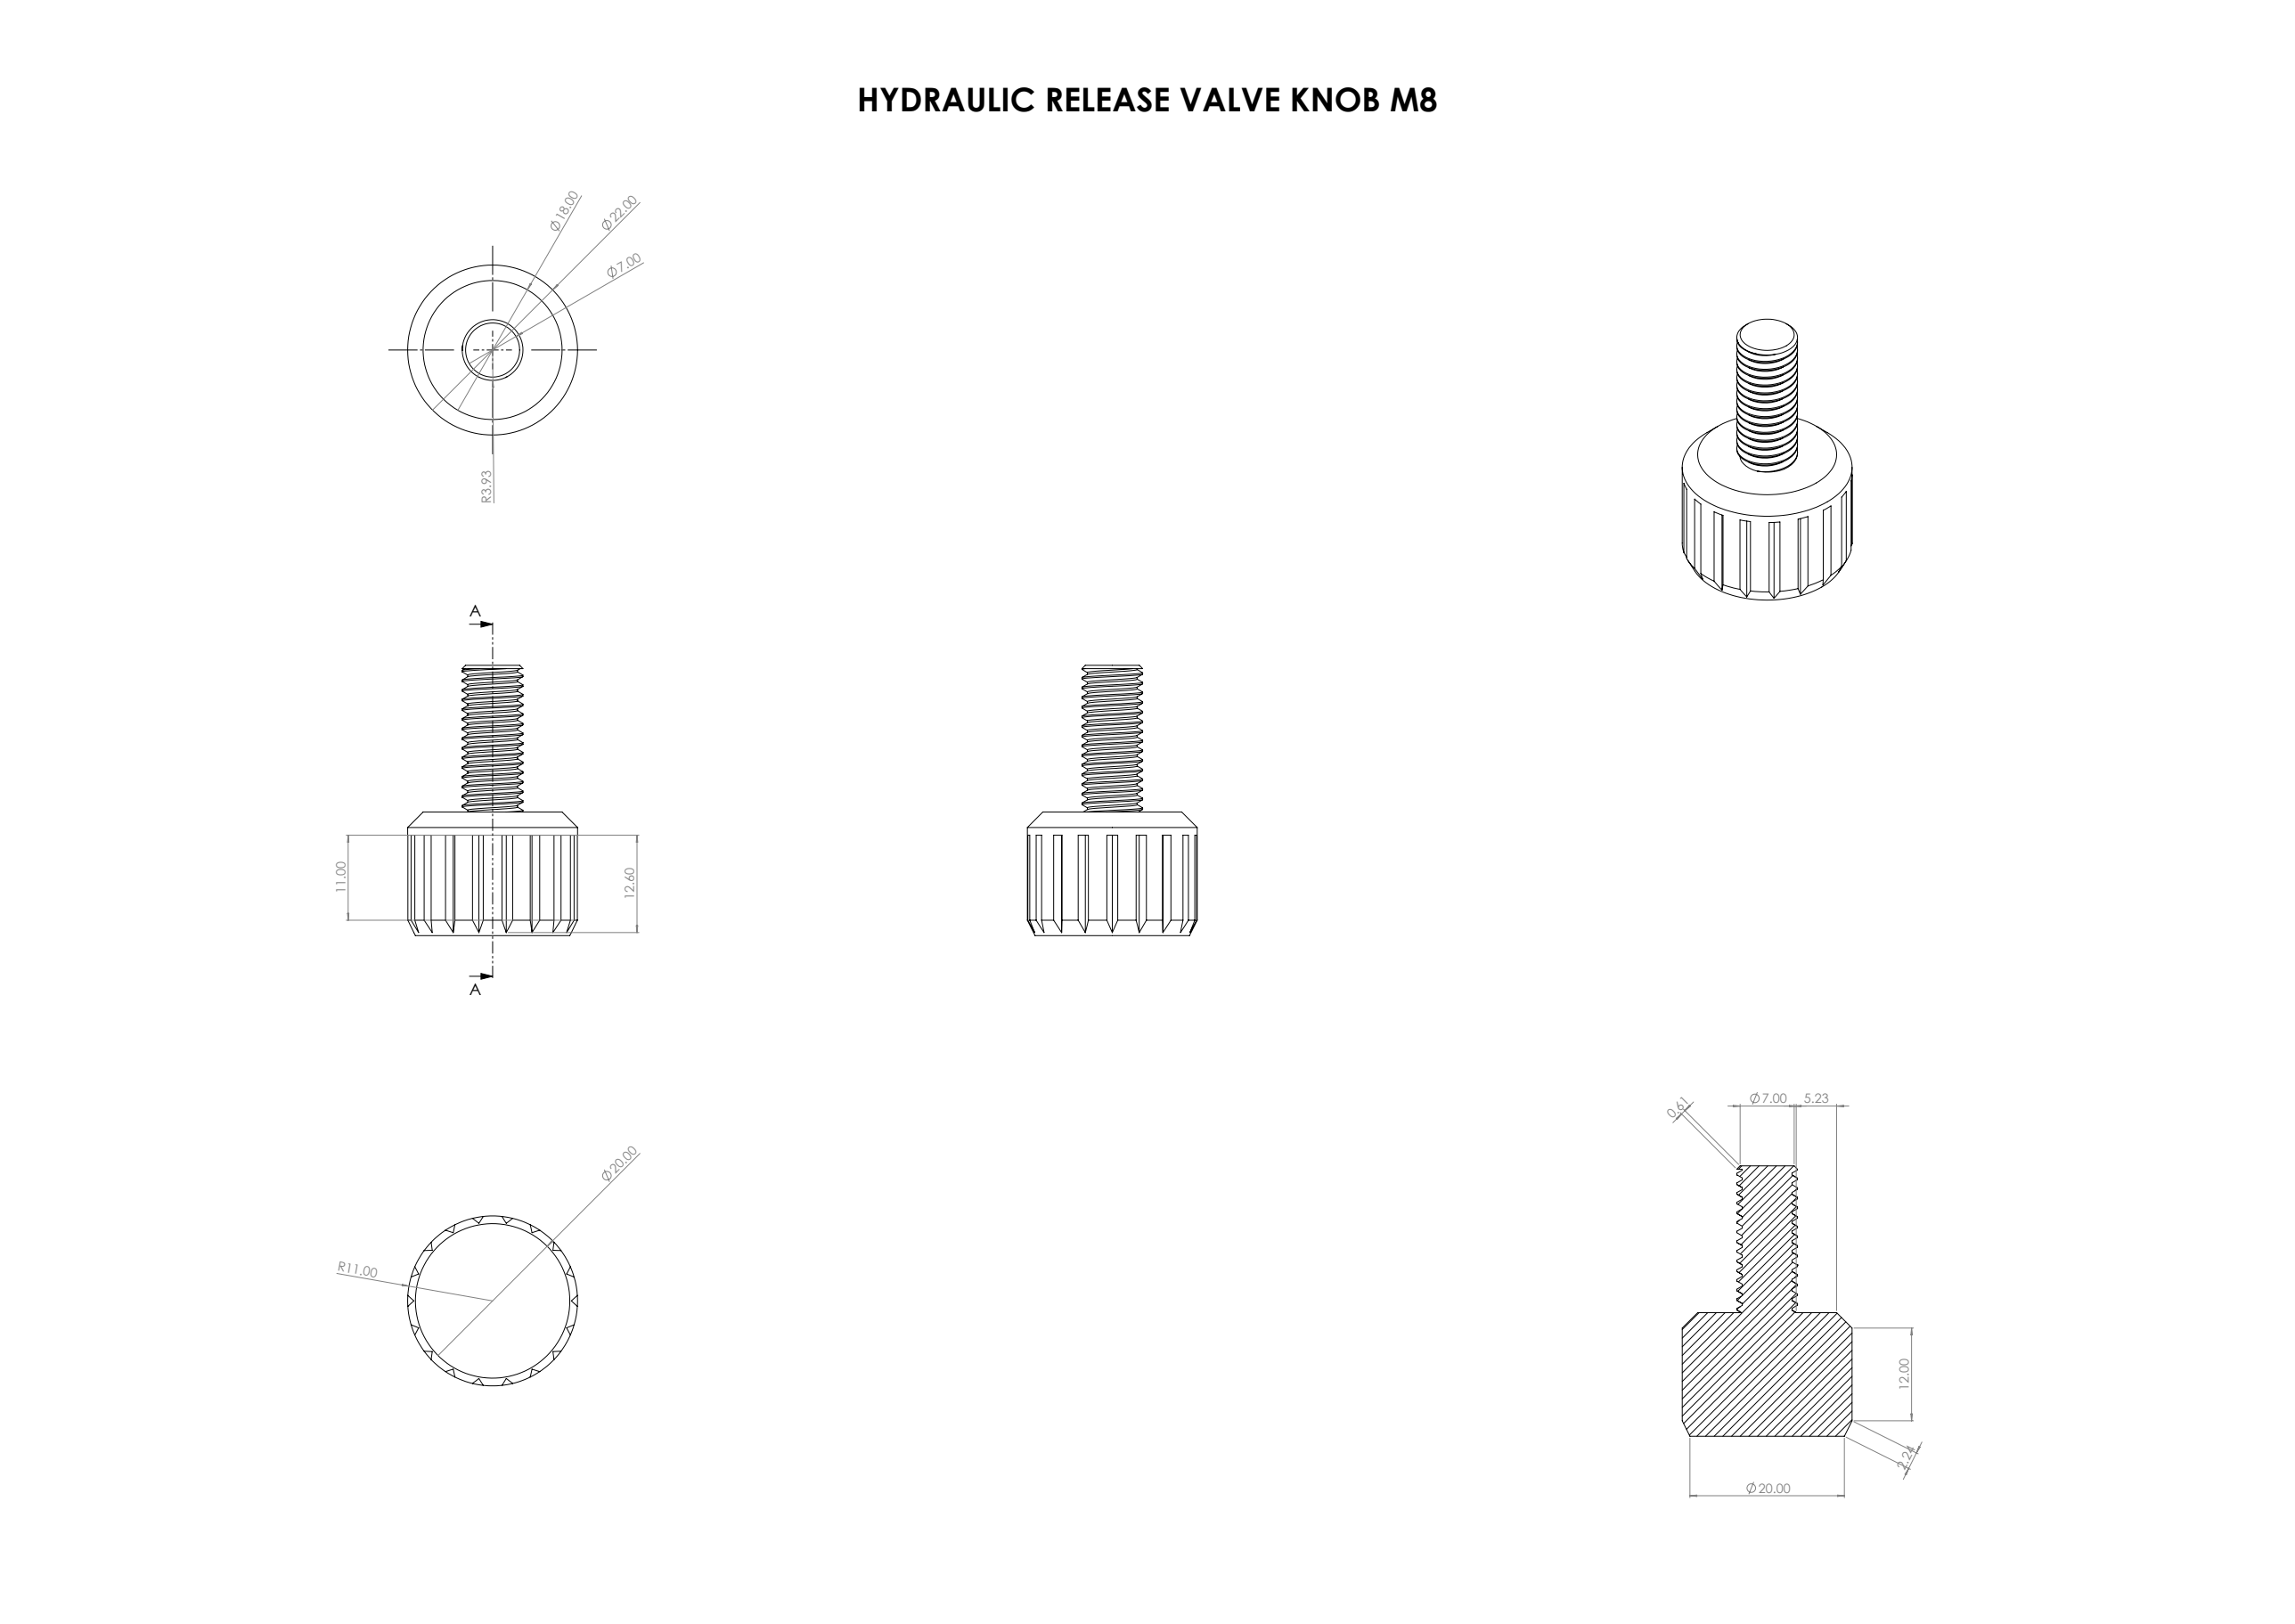
ISO-10303-21;
HEADER;
/* Generated by software containing ST-Developer
 * from STEP Tools, Inc. (www.steptools.com) 
 */

FILE_DESCRIPTION(
/* description */ (''),
/* implementation_level */ '2;1');

FILE_NAME(
/* name */ '12_Hydraulic_Release_Valve_Knob_M8.step',
/* time_stamp */ '2026-10-20T10:03:03-07:00',
/* author */ (''),
/* organization */ (''),
/* preprocessor_version */ 'ST-DEVELOPER v20.2',
/* originating_system */ 'Autodesk Translation Framework v15.15.0.0',
/* authorisation */ '');

FILE_SCHEMA (('AUTOMOTIVE_DESIGN { 1 0 10303 214 3 1 1 }'));
ENDSEC;

DATA;
#10=MECHANICAL_DESIGN_GEOMETRIC_PRESENTATION_REPRESENTATION('',(#530),#71492);
#319=(
BOUNDED_CURVE()
B_SPLINE_CURVE(2,(#47148,#47149,#47150),.UNSPECIFIED.,.F.,.F.)
B_SPLINE_CURVE_WITH_KNOTS((3,3),(0.0512618960218088,0.239747982802954),
 .UNSPECIFIED.)
CURVE()
GEOMETRIC_REPRESENTATION_ITEM()
RATIONAL_B_SPLINE_CURVE((1.0006680999084,1.00156232618943,1.))
REPRESENTATION_ITEM('')
);
#320=(
BOUNDED_CURVE()
B_SPLINE_CURVE(2,(#47162,#47163,#47164),.UNSPECIFIED.,.F.,.F.)
B_SPLINE_CURVE_WITH_KNOTS((3,3),(0.,0.18848608678106),.UNSPECIFIED.)
CURVE()
GEOMETRIC_REPRESENTATION_ITEM()
RATIONAL_B_SPLINE_CURVE((1.,1.0015623261938,1.00066809991027))
REPRESENTATION_ITEM('')
);
#321=(
BOUNDED_CURVE()
B_SPLINE_CURVE(2,(#47169,#47170,#47171),.UNSPECIFIED.,.F.,.F.)
B_SPLINE_CURVE_WITH_KNOTS((3,3),(0.0512618960217405,0.239747982802953),
 .UNSPECIFIED.)
CURVE()
GEOMETRIC_REPRESENTATION_ITEM()
RATIONAL_B_SPLINE_CURVE((1.00066809990968,1.00156232619242,1.))
REPRESENTATION_ITEM('')
);
#322=(
BOUNDED_CURVE()
B_SPLINE_CURVE(2,(#47183,#47184,#47185),.UNSPECIFIED.,.F.,.F.)
B_SPLINE_CURVE_WITH_KNOTS((3,3),(0.,0.188486086781626),.UNSPECIFIED.)
CURVE()
GEOMETRIC_REPRESENTATION_ITEM()
RATIONAL_B_SPLINE_CURVE((1.,1.00156232620375,1.00066809991451))
REPRESENTATION_ITEM('')
);
#323=(
BOUNDED_CURVE()
B_SPLINE_CURVE(2,(#47190,#47191,#47192),.UNSPECIFIED.,.F.,.F.)
B_SPLINE_CURVE_WITH_KNOTS((3,3),(0.051261896021783,0.239747982802949),
 .UNSPECIFIED.)
CURVE()
GEOMETRIC_REPRESENTATION_ITEM()
RATIONAL_B_SPLINE_CURVE((1.0006680999091,1.00156232619108,1.))
REPRESENTATION_ITEM('')
);
#324=(
BOUNDED_CURVE()
B_SPLINE_CURVE(2,(#47204,#47205,#47206),.UNSPECIFIED.,.F.,.F.)
B_SPLINE_CURVE_WITH_KNOTS((3,3),(0.,0.188486086780641),.UNSPECIFIED.)
CURVE()
GEOMETRIC_REPRESENTATION_ITEM()
RATIONAL_B_SPLINE_CURVE((1.,1.00156232617076,1.00066809990042))
REPRESENTATION_ITEM('')
);
#325=(
BOUNDED_CURVE()
B_SPLINE_CURVE(2,(#47211,#47212,#47213),.UNSPECIFIED.,.F.,.F.)
B_SPLINE_CURVE_WITH_KNOTS((3,3),(0.0512618960212928,0.239747982802966),
 .UNSPECIFIED.)
CURVE()
GEOMETRIC_REPRESENTATION_ITEM()
RATIONAL_B_SPLINE_CURVE((1.00066809991313,1.0015623262005,1.))
REPRESENTATION_ITEM('')
);
#326=(
BOUNDED_CURVE()
B_SPLINE_CURVE(2,(#47225,#47226,#47227),.UNSPECIFIED.,.F.,.F.)
B_SPLINE_CURVE_WITH_KNOTS((3,3),(0.,0.18848608678103),.UNSPECIFIED.)
CURVE()
GEOMETRIC_REPRESENTATION_ITEM()
RATIONAL_B_SPLINE_CURVE((1.,1.00156232618489,1.00066809990646))
REPRESENTATION_ITEM('')
);
#327=(
BOUNDED_CURVE()
B_SPLINE_CURVE(2,(#47232,#47233,#47234),.UNSPECIFIED.,.F.,.F.)
B_SPLINE_CURVE_WITH_KNOTS((3,3),(0.0512618960214512,0.239747982802948),
 .UNSPECIFIED.)
CURVE()
GEOMETRIC_REPRESENTATION_ITEM()
RATIONAL_B_SPLINE_CURVE((1.00066809991422,1.00156232620306,1.))
REPRESENTATION_ITEM('')
);
#328=(
BOUNDED_CURVE()
B_SPLINE_CURVE(2,(#47246,#47247,#47248),.UNSPECIFIED.,.F.,.F.)
B_SPLINE_CURVE_WITH_KNOTS((3,3),(0.,0.188486086781497),.UNSPECIFIED.)
CURVE()
GEOMETRIC_REPRESENTATION_ITEM()
RATIONAL_B_SPLINE_CURVE((1.,1.00156232620306,1.00066809991422))
REPRESENTATION_ITEM('')
);
#329=(
BOUNDED_CURVE()
B_SPLINE_CURVE(2,(#47253,#47254,#47255),.UNSPECIFIED.,.F.,.F.)
B_SPLINE_CURVE_WITH_KNOTS((3,3),(0.0512618960218087,0.239747982802954),
 .UNSPECIFIED.)
CURVE()
GEOMETRIC_REPRESENTATION_ITEM()
RATIONAL_B_SPLINE_CURVE((1.0006680999084,1.00156232618943,1.))
REPRESENTATION_ITEM('')
);
#330=(
BOUNDED_CURVE()
B_SPLINE_CURVE(2,(#47267,#47268,#47269),.UNSPECIFIED.,.F.,.F.)
B_SPLINE_CURVE_WITH_KNOTS((3,3),(0.,0.188486086780909),.UNSPECIFIED.)
CURVE()
GEOMETRIC_REPRESENTATION_ITEM()
RATIONAL_B_SPLINE_CURVE((1.,1.00156232618876,1.00066809990812))
REPRESENTATION_ITEM('')
);
#331=(
BOUNDED_CURVE()
B_SPLINE_CURVE(2,(#47274,#47275,#47276),.UNSPECIFIED.,.F.,.F.)
B_SPLINE_CURVE_WITH_KNOTS((3,3),(0.0512618960214397,0.239747982802953),
 .UNSPECIFIED.)
CURVE()
GEOMETRIC_REPRESENTATION_ITEM()
RATIONAL_B_SPLINE_CURVE((1.00066809991433,1.00156232620331,1.))
REPRESENTATION_ITEM('')
);
#332=(
BOUNDED_CURVE()
B_SPLINE_CURVE(2,(#47288,#47289,#47290),.UNSPECIFIED.,.F.,.F.)
B_SPLINE_CURVE_WITH_KNOTS((3,3),(0.,0.188486086781649),.UNSPECIFIED.)
CURVE()
GEOMETRIC_REPRESENTATION_ITEM()
RATIONAL_B_SPLINE_CURVE((1.,1.00156232620001,1.00066809991291))
REPRESENTATION_ITEM('')
);
#333=(
BOUNDED_CURVE()
B_SPLINE_CURVE(2,(#47295,#47296,#47297),.UNSPECIFIED.,.F.,.F.)
B_SPLINE_CURVE_WITH_KNOTS((3,3),(0.0512618960219227,0.239747982802949),
 .UNSPECIFIED.)
CURVE()
GEOMETRIC_REPRESENTATION_ITEM()
RATIONAL_B_SPLINE_CURVE((1.00066809990695,1.00156232618604,1.))
REPRESENTATION_ITEM('')
);
#334=(
BOUNDED_CURVE()
B_SPLINE_CURVE(2,(#47309,#47310,#47311),.UNSPECIFIED.,.F.,.F.)
B_SPLINE_CURVE_WITH_KNOTS((3,3),(0.,0.188486086780641),.UNSPECIFIED.)
CURVE()
GEOMETRIC_REPRESENTATION_ITEM()
RATIONAL_B_SPLINE_CURVE((1.,1.00156232617076,1.00066809990042))
REPRESENTATION_ITEM('')
);
#335=(
BOUNDED_CURVE()
B_SPLINE_CURVE(2,(#47316,#47317,#47318),.UNSPECIFIED.,.F.,.F.)
B_SPLINE_CURVE_WITH_KNOTS((3,3),(0.0512618960215005,0.239747982802966),
 .UNSPECIFIED.)
CURVE()
GEOMETRIC_REPRESENTATION_ITEM()
RATIONAL_B_SPLINE_CURVE((1.00066809990987,1.00156232619288,1.))
REPRESENTATION_ITEM('')
);
#336=(
BOUNDED_CURVE()
B_SPLINE_CURVE(2,(#47330,#47331,#47332),.UNSPECIFIED.,.F.,.F.)
B_SPLINE_CURVE_WITH_KNOTS((3,3),(0.,0.188486086781019),.UNSPECIFIED.)
CURVE()
GEOMETRIC_REPRESENTATION_ITEM()
RATIONAL_B_SPLINE_CURVE((1.,1.00156232618454,1.00066809990631))
REPRESENTATION_ITEM('')
);
#337=(
BOUNDED_CURVE()
B_SPLINE_CURVE(2,(#47337,#47338,#47339),.UNSPECIFIED.,.F.,.F.)
B_SPLINE_CURVE_WITH_KNOTS((3,3),(0.0512618960218745,0.239747982802939),
 .UNSPECIFIED.)
CURVE()
GEOMETRIC_REPRESENTATION_ITEM()
RATIONAL_B_SPLINE_CURVE((1.00066809991027,1.0015623261938,1.))
REPRESENTATION_ITEM('')
);
#338=(
BOUNDED_CURVE()
B_SPLINE_CURVE(2,(#47351,#47352,#47353),.UNSPECIFIED.,.F.,.F.)
B_SPLINE_CURVE_WITH_KNOTS((3,3),(0.,0.188486086781156),.UNSPECIFIED.)
CURVE()
GEOMETRIC_REPRESENTATION_ITEM()
RATIONAL_B_SPLINE_CURVE((1.,1.00156232618832,1.00066809990792))
REPRESENTATION_ITEM('')
);
#339=(
BOUNDED_CURVE()
B_SPLINE_CURVE(2,(#47358,#47359,#47360),.UNSPECIFIED.,.F.,.F.)
B_SPLINE_CURVE_WITH_KNOTS((3,3),(0.0512618960213807,0.239747982802952),
 .UNSPECIFIED.)
CURVE()
GEOMETRIC_REPRESENTATION_ITEM()
RATIONAL_B_SPLINE_CURVE((1.00066809991545,1.00156232620592,1.))
REPRESENTATION_ITEM('')
);
#340=(
BOUNDED_CURVE()
B_SPLINE_CURVE(2,(#47372,#47373,#47374),.UNSPECIFIED.,.F.,.F.)
B_SPLINE_CURVE_WITH_KNOTS((3,3),(0.,0.188486086781477),.UNSPECIFIED.)
CURVE()
GEOMETRIC_REPRESENTATION_ITEM()
RATIONAL_B_SPLINE_CURVE((1.,1.0015623262088,1.00066809991668))
REPRESENTATION_ITEM('')
);
#341=(
BOUNDED_CURVE()
B_SPLINE_CURVE(2,(#47379,#47380,#47381),.UNSPECIFIED.,.F.,.F.)
B_SPLINE_CURVE_WITH_KNOTS((3,3),(0.0512618960223282,0.239747982802951),
 .UNSPECIFIED.)
CURVE()
GEOMETRIC_REPRESENTATION_ITEM()
RATIONAL_B_SPLINE_CURVE((1.00066809990016,1.00156232617014,1.))
REPRESENTATION_ITEM('')
);
#342=(
BOUNDED_CURVE()
B_SPLINE_CURVE(2,(#47393,#47394,#47395),.UNSPECIFIED.,.F.,.F.)
B_SPLINE_CURVE_WITH_KNOTS((3,3),(0.,0.188486086781308),.UNSPECIFIED.)
CURVE()
GEOMETRIC_REPRESENTATION_ITEM()
RATIONAL_B_SPLINE_CURVE((1.,1.00156232619586,1.00066809991115))
REPRESENTATION_ITEM('')
);
#343=(
BOUNDED_CURVE()
B_SPLINE_CURVE(2,(#47400,#47401,#47402),.UNSPECIFIED.,.F.,.F.)
B_SPLINE_CURVE_WITH_KNOTS((3,3),(0.051261896021939,0.239747982802949),
 .UNSPECIFIED.)
CURVE()
GEOMETRIC_REPRESENTATION_ITEM()
RATIONAL_B_SPLINE_CURVE((1.00066809990618,1.00156232618425,1.))
REPRESENTATION_ITEM('')
);
#344=(
BOUNDED_CURVE()
B_SPLINE_CURVE(2,(#47414,#47415,#47416),.UNSPECIFIED.,.F.,.F.)
B_SPLINE_CURVE_WITH_KNOTS((3,3),(0.,0.188486086781416),.UNSPECIFIED.)
CURVE()
GEOMETRIC_REPRESENTATION_ITEM()
RATIONAL_B_SPLINE_CURVE((1.,1.0015623261913,1.0006680999092))
REPRESENTATION_ITEM('')
);
#345=(
BOUNDED_CURVE()
B_SPLINE_CURVE(2,(#47421,#47422,#47423),.UNSPECIFIED.,.F.,.F.)
B_SPLINE_CURVE_WITH_KNOTS((3,3),(0.0512618960214561,0.239747982802948),
 .UNSPECIFIED.)
CURVE()
GEOMETRIC_REPRESENTATION_ITEM()
RATIONAL_B_SPLINE_CURVE((1.00066809991424,1.00156232620311,1.))
REPRESENTATION_ITEM('')
);
#346=(
BOUNDED_CURVE()
B_SPLINE_CURVE(2,(#47437,#47438,#47439),.UNSPECIFIED.,.F.,.F.)
B_SPLINE_CURVE_WITH_KNOTS((3,3),(0.,0.188486086781106),.UNSPECIFIED.)
CURVE()
GEOMETRIC_REPRESENTATION_ITEM()
RATIONAL_B_SPLINE_CURVE((1.,1.00156232618923,1.00066809990831))
REPRESENTATION_ITEM('')
);
#347=(
BOUNDED_CURVE()
B_SPLINE_CURVE(2,(#47444,#47445,#47446),.UNSPECIFIED.,.F.,.F.)
B_SPLINE_CURVE_WITH_KNOTS((3,3),(0.0512618960218789,0.239747982802938),
 .UNSPECIFIED.)
CURVE()
GEOMETRIC_REPRESENTATION_ITEM()
RATIONAL_B_SPLINE_CURVE((1.00066809991027,1.0015623261938,1.))
REPRESENTATION_ITEM('')
);
#348=(
BOUNDED_CURVE()
B_SPLINE_CURVE(2,(#47458,#47459,#47460),.UNSPECIFIED.,.F.,.F.)
B_SPLINE_CURVE_WITH_KNOTS((3,3),(0.,0.188486086781156),.UNSPECIFIED.)
CURVE()
GEOMETRIC_REPRESENTATION_ITEM()
RATIONAL_B_SPLINE_CURVE((1.,1.00156232618832,1.00066809990792))
REPRESENTATION_ITEM('')
);
#349=(
BOUNDED_CURVE()
B_SPLINE_CURVE(2,(#47465,#47466,#47467),.UNSPECIFIED.,.F.,.F.)
B_SPLINE_CURVE_WITH_KNOTS((3,3),(0.0512618960211266,0.239747982802957),
 .UNSPECIFIED.)
CURVE()
GEOMETRIC_REPRESENTATION_ITEM()
RATIONAL_B_SPLINE_CURVE((1.00066809991756,1.00156232621087,1.))
REPRESENTATION_ITEM('')
);
#350=(
BOUNDED_CURVE()
B_SPLINE_CURVE(2,(#47479,#47480,#47481),.UNSPECIFIED.,.F.,.F.)
B_SPLINE_CURVE_WITH_KNOTS((3,3),(0.,0.188486086781475),.UNSPECIFIED.)
CURVE()
GEOMETRIC_REPRESENTATION_ITEM()
RATIONAL_B_SPLINE_CURVE((1.,1.0015623262088,1.00066809991668))
REPRESENTATION_ITEM('')
);
#351=(
BOUNDED_CURVE()
B_SPLINE_CURVE(2,(#47486,#47487,#47488),.UNSPECIFIED.,.F.,.F.)
B_SPLINE_CURVE_WITH_KNOTS((3,3),(0.0512618960222505,0.239747982802951),
 .UNSPECIFIED.)
CURVE()
GEOMETRIC_REPRESENTATION_ITEM()
RATIONAL_B_SPLINE_CURVE((1.00066809990131,1.00156232617284,1.))
REPRESENTATION_ITEM('')
);
#352=(
BOUNDED_CURVE()
B_SPLINE_CURVE(2,(#47500,#47501,#47502),.UNSPECIFIED.,.F.,.F.)
B_SPLINE_CURVE_WITH_KNOTS((3,3),(0.,0.188486086781171),.UNSPECIFIED.)
CURVE()
GEOMETRIC_REPRESENTATION_ITEM()
RATIONAL_B_SPLINE_CURVE((1.,1.00156232619143,1.00066809990925))
REPRESENTATION_ITEM('')
);
#353=(
BOUNDED_CURVE()
B_SPLINE_CURVE(2,(#47507,#47508,#47509),.UNSPECIFIED.,.F.,.F.)
B_SPLINE_CURVE_WITH_KNOTS((3,3),(0.0512618960219306,0.239747982802949),
 .UNSPECIFIED.)
CURVE()
GEOMETRIC_REPRESENTATION_ITEM()
RATIONAL_B_SPLINE_CURVE((1.00066809990631,1.00156232618454,1.))
REPRESENTATION_ITEM('')
);
#354=(
BOUNDED_CURVE()
B_SPLINE_CURVE(2,(#47521,#47522,#47523),.UNSPECIFIED.,.F.,.F.)
B_SPLINE_CURVE_WITH_KNOTS((3,3),(0.,0.188486086781674),.UNSPECIFIED.)
CURVE()
GEOMETRIC_REPRESENTATION_ITEM()
RATIONAL_B_SPLINE_CURVE((1.,1.0015623262005,1.00066809991312))
REPRESENTATION_ITEM('')
);
#388=SHAPE_REPRESENTATION_RELATIONSHIP('SRR','None',#71609,#407);
#407=ADVANCED_BREP_SHAPE_REPRESENTATION('',(#426),#71479);
#426=MANIFOLD_SOLID_BREP('Release knob',#28465);
#530=STYLED_ITEM('',(#71873),#426);
#810=B_SPLINE_CURVE_WITH_KNOTS('',3,(#46072,#46073,#46074,#46075,#46076,
#46077,#46078,#46079,#46080,#46081),.UNSPECIFIED.,.F.,.F.,(4,3,3,4),(-4.09274904019441,
-3.97454678650995,-2.98091008988247,-2.06120159751572),.UNSPECIFIED.);
#811=B_SPLINE_CURVE_WITH_KNOTS('',3,(#46084,#46085,#46086,#46087,#46088,
#46089,#46090,#46091,#46092,#46093),.UNSPECIFIED.,.F.,.F.,(4,3,3,4),(0.,
0.496818348313743,0.993636696627499,1.11004521091142),.UNSPECIFIED.);
#812=B_SPLINE_CURVE_WITH_KNOTS('',3,(#46098,#46099,#46100,#46101,#46102,
#46103,#46104,#46105,#46106,#46107,#46108,#46109,#46110,#46111,#46112,#46113,
#46114,#46115,#46116,#46117,#46118,#46119),.UNSPECIFIED.,.F.,.F.,(4,3,3,
3,3,3,3,4),(-10.375934347374,-9.93636696627486,-8.94273026964737,-7.94909357301989,
-6.9554568763924,-5.96182017976492,-4.96818348313743,-4.09274904019441),
 .UNSPECIFIED.);
#813=B_SPLINE_CURVE_WITH_KNOTS('',3,(#46120,#46121,#46122,#46123,#46124,
#46125,#46126,#46127,#46128,#46129,#46130,#46131,#46132,#46133,#46134,#46135,
#46136,#46137,#46138,#46139,#46140,#46141),.UNSPECIFIED.,.F.,.F.,(4,3,3,
3,3,3,3,4),(1.11004521091142,1.98727339325499,2.98091008988248,3.97454678650997,
4.96818348313745,5.96182017976494,6.95545687639243,7.393230518091),
 .UNSPECIFIED.);
#814=B_SPLINE_CURVE_WITH_KNOTS('',3,(#46146,#46147,#46148,#46149,#46150,
#46151,#46152,#46153,#46154,#46155,#46156,#46157,#46158,#46159,#46160,#46161,
#46162,#46163,#46164,#46165,#46166,#46167),.UNSPECIFIED.,.F.,.F.,(4,3,3,
3,3,3,3,4),(-16.6591196545536,-15.8981871460398,-14.9045504494123,-13.9109137527848,
-12.9172770561573,-11.9236403595298,-10.9300036629023,-10.375934347374),
 .UNSPECIFIED.);
#815=B_SPLINE_CURVE_WITH_KNOTS('',3,(#46168,#46169,#46170,#46171,#46172,
#46173,#46174,#46175,#46176,#46177,#46178,#46179,#46180,#46181,#46182,#46183,
#46184,#46185,#46186,#46187,#46188,#46189),.UNSPECIFIED.,.F.,.F.,(4,3,3,
3,3,3,3,4),(7.393230518091,7.94909357301991,8.94273026964739,9.93636696627487,
10.9300036629024,11.9236403595298,12.9172770561573,13.6764158252706),
 .UNSPECIFIED.);
#816=B_SPLINE_CURVE_WITH_KNOTS('',3,(#46194,#46195,#46196,#46197,#46198,
#46199,#46200,#46201,#46202,#46203,#46204,#46205,#46206,#46207,#46208,#46209,
#46210,#46211,#46212,#46213,#46214,#46215,#46216,#46217,#46218),
 .UNSPECIFIED.,.F.,.F.,(4,3,3,3,3,3,3,3,4),(-22.9423049617332,-22.8536440224322,
-21.8600073258047,-20.8663706291772,-19.8727339325497,-18.8790972359222,
-17.8854605392947,-16.8918238426673,-16.6591196545536),.UNSPECIFIED.);
#817=B_SPLINE_CURVE_WITH_KNOTS('',3,(#46219,#46220,#46221,#46222,#46223,
#46224,#46225,#46226,#46227,#46228,#46229,#46230,#46231,#46232,#46233,#46234,
#46235,#46236,#46237,#46238,#46239,#46240,#46241,#46242,#46243),
 .UNSPECIFIED.,.F.,.F.,(4,3,3,3,3,3,3,3,4),(13.6764158252706,13.9109137527848,
14.9045504494123,15.8981871460398,16.8918238426673,17.8854605392947,18.8790972359222,
19.8727339325497,19.9596011324502),.UNSPECIFIED.);
#818=B_SPLINE_CURVE_WITH_KNOTS('',3,(#46248,#46249,#46250,#46251,#46252,
#46253,#46254,#46255,#46256,#46257,#46258,#46259,#46260,#46261,#46262,#46263,
#46264,#46265,#46266,#46267,#46268,#46269),.UNSPECIFIED.,.F.,.F.,(4,3,3,
3,3,3,3,4),(-29.2254902689127,-28.8154642021971,-27.8218275055696,-26.8281908089421,
-25.8345541123146,-24.8409174156871,-23.8472807190597,-22.9423049617332),
 .UNSPECIFIED.);
#819=B_SPLINE_CURVE_WITH_KNOTS('',3,(#46270,#46271,#46272,#46273,#46274,
#46275,#46276,#46277,#46278,#46279,#46280,#46281,#46282,#46283,#46284,#46285,
#46286,#46287,#46288,#46289,#46290,#46291),.UNSPECIFIED.,.F.,.F.,(4,3,3,
3,3,3,3,4),(19.9596011324502,20.8663706291772,21.8600073258047,22.8536440224322,
23.8472807190597,24.8409174156871,25.8345541123146,26.2427864396298),
 .UNSPECIFIED.);
#820=B_SPLINE_CURVE_WITH_KNOTS('',3,(#46296,#46297,#46298,#46299,#46300,
#46301,#46302,#46303,#46304,#46305,#46306,#46307,#46308,#46309,#46310,#46311,
#46312,#46313,#46314,#46315,#46316,#46317),.UNSPECIFIED.,.F.,.F.,(4,3,3,
3,3,3,3,4),(-35.5086755760923,-34.777284381962,-33.7836476853345,-32.790010988707,
-31.7963742920795,-30.802737595452,-29.8091008988246,-29.2254902689127),
 .UNSPECIFIED.);
#821=B_SPLINE_CURVE_WITH_KNOTS('',3,(#46318,#46319,#46320,#46321,#46322,
#46323,#46324,#46325,#46326,#46327,#46328,#46329,#46330,#46331,#46332,#46333,
#46334,#46335,#46336,#46337,#46338,#46339),.UNSPECIFIED.,.F.,.F.,(4,3,3,
3,3,3,3,4),(26.2427864396298,26.8281908089421,27.8218275055696,28.8154642021971,
29.8091008988246,30.8027375954521,31.7963742920795,32.5259717468093),
 .UNSPECIFIED.);
#822=B_SPLINE_CURVE_WITH_KNOTS('',3,(#46344,#46345,#46346,#46347,#46348,
#46349,#46350,#46351,#46352,#46353,#46354,#46355,#46356,#46357,#46358,#46359,
#46360,#46361,#46362,#46363,#46364,#46365,#46366,#46367,#46368),
 .UNSPECIFIED.,.F.,.F.,(4,3,3,3,3,3,3,3,4),(-41.7918608832719,-41.7327412583544,
-40.7391045617269,-39.7454678650994,-38.7518311684719,-37.7581944718444,
-36.764557775217,-35.7709210785895,-35.5086755760923),.UNSPECIFIED.);
#823=B_SPLINE_CURVE_WITH_KNOTS('',3,(#46369,#46370,#46371,#46372,#46373,
#46374,#46375,#46376,#46377,#46378,#46379,#46380,#46381,#46382,#46383,#46384,
#46385,#46386,#46387,#46388,#46389,#46390,#46391,#46392,#46393),
 .UNSPECIFIED.,.F.,.F.,(4,3,3,3,3,3,3,3,4),(32.5259717468093,32.790010988707,
33.7836476853345,34.777284381962,35.7709210785895,36.764557775217,37.7581944718445,
38.751831168472,38.8091570539889),.UNSPECIFIED.);
#824=B_SPLINE_CURVE_WITH_KNOTS('',3,(#46398,#46399,#46400,#46401,#46402,
#46403,#46404,#46405,#46406,#46407,#46408,#46409,#46410,#46411,#46412,#46413,
#46414,#46415,#46416,#46417,#46418,#46419),.UNSPECIFIED.,.F.,.F.,(4,3,3,
3,3,3,3,4),(-48.0750461904515,-47.6945614381193,-46.7009247414918,-45.7072880448643,
-44.7136513482368,-43.7200146516094,-42.7263779549819,-41.7918608832719),
 .UNSPECIFIED.);
#825=B_SPLINE_CURVE_WITH_KNOTS('',3,(#46420,#46421,#46422,#46423,#46424,
#46425,#46426,#46427,#46428,#46429,#46430,#46431,#46432,#46433,#46434,#46435,
#46436,#46437,#46438,#46439,#46440,#46441),.UNSPECIFIED.,.F.,.F.,(4,3,3,
3,3,3,3,4),(38.8091570539889,39.7454678650994,40.7391045617269,41.7327412583544,
42.7263779549819,43.7200146516094,44.7136513482369,45.0923423611685),
 .UNSPECIFIED.);
#826=B_SPLINE_CURVE_WITH_KNOTS('',3,(#46446,#46447,#46448,#46449,#46450,
#46451,#46452,#46453,#46454,#46455,#46456,#46457,#46458,#46459,#46460,#46461,
#46462,#46463,#46464,#46465,#46466,#46467),.UNSPECIFIED.,.F.,.F.,(4,3,3,
3,3,3,3,4),(-54.3582314976311,-53.6563816178842,-52.6627449212567,-51.6691082246292,
-50.6754715280018,-49.6818348313743,-48.6881981347468,-48.0750461904515),
 .UNSPECIFIED.);
#827=B_SPLINE_CURVE_WITH_KNOTS('',3,(#46468,#46469,#46470,#46471,#46472,
#46473,#46474,#46475,#46476,#46477,#46478,#46479,#46480,#46481,#46482,#46483,
#46484,#46485,#46486,#46487,#46488,#46489),.UNSPECIFIED.,.F.,.F.,(4,3,3,
3,3,3,3,4),(45.0923423611685,45.7072880448643,46.7009247414918,47.6945614381193,
48.6881981347468,49.6818348313743,50.6754715280018,51.3755276683481),
 .UNSPECIFIED.);
#828=B_SPLINE_CURVE_WITH_KNOTS('',3,(#46494,#46495,#46496,#46497,#46498,
#46499,#46500,#46501,#46502,#46503,#46504,#46505,#46506,#46507,#46508,#46509,
#46510,#46511,#46512,#46513,#46514,#46515,#46516,#46517,#46518),
 .UNSPECIFIED.,.F.,.F.,(4,3,3,3,3,3,3,3,4),(-60.6414168048107,-60.6118384942766,
-59.6182017976491,-58.6245651010216,-57.6309284043942,-56.6372917077667,
-55.6436550111392,-54.6500183145117,-54.3582314976311),.UNSPECIFIED.);
#829=B_SPLINE_CURVE_WITH_KNOTS('',3,(#46519,#46520,#46521,#46522,#46523,
#46524,#46525,#46526,#46527,#46528,#46529,#46530,#46531,#46532,#46533,#46534,
#46535,#46536,#46537,#46538,#46539,#46540,#46541,#46542,#46543),
 .UNSPECIFIED.,.F.,.F.,(4,3,3,3,3,3,3,3,4),(51.3755276683481,51.6691082246293,
52.6627449212567,53.6563816178842,54.6500183145117,55.6436550111392,56.6372917077667,
57.6309284043942,57.6587129755277),.UNSPECIFIED.);
#830=B_SPLINE_CURVE_WITH_KNOTS('',3,(#46548,#46549,#46550,#46551,#46552,
#46553,#46554,#46555,#46556,#46557,#46558,#46559,#46560,#46561,#46562,#46563,
#46564,#46565,#46566,#46567,#46568,#46569),.UNSPECIFIED.,.F.,.F.,(4,3,3,
3,3,3,3,4),(-66.9246021119903,-66.5736586740415,-65.580021977414,-64.5863852807866,
-63.5927485841591,-62.5991118875316,-61.6054751909041,-60.6414168048107),
 .UNSPECIFIED.);
#831=B_SPLINE_CURVE_WITH_KNOTS('',3,(#46570,#46571,#46572,#46573,#46574,
#46575,#46576,#46577,#46578,#46579,#46580,#46581,#46582,#46583,#46584,#46585,
#46586,#46587,#46588,#46589,#46590,#46591),.UNSPECIFIED.,.F.,.F.,(4,3,3,
3,3,3,3,4),(57.6587129755277,58.6245651010217,59.6182017976491,60.6118384942766,
61.6054751909041,62.5991118875316,63.5927485841591,63.9418982827073),
 .UNSPECIFIED.);
#832=B_SPLINE_CURVE_WITH_KNOTS('',3,(#46596,#46597,#46598,#46599,#46600,
#46601,#46602,#46603,#46604,#46605,#46606,#46607,#46608,#46609,#46610,#46611,
#46612,#46613,#46614,#46615,#46616,#46617),.UNSPECIFIED.,.F.,.F.,(4,3,3,
3,3,3,3,4),(-73.2077874191699,-72.5354788538064,-71.541842157179,-70.5482054605515,
-69.554568763924,-68.5609320672965,-67.567295370669,-66.9246021119903),
 .UNSPECIFIED.);
#833=B_SPLINE_CURVE_WITH_KNOTS('',3,(#46618,#46619,#46620,#46621,#46622,
#46623,#46624,#46625,#46626,#46627,#46628,#46629,#46630,#46631,#46632,#46633,
#46634,#46635,#46636,#46637,#46638,#46639),.UNSPECIFIED.,.F.,.F.,(4,3,3,
3,3,3,3,4),(63.9418982827073,64.5863852807866,65.580021977414,66.5736586740415,
67.567295370669,68.5609320672965,69.554568763924,70.2250835898869),
 .UNSPECIFIED.);
#834=B_SPLINE_CURVE_WITH_KNOTS('',3,(#46644,#46645,#46646,#46647,#46648,
#46649,#46650,#46651,#46652,#46653,#46654,#46655,#46656,#46657,#46658,#46659,
#46660,#46661,#46662,#46663,#46664,#46665),.UNSPECIFIED.,.F.,.F.,(4,3,3,
3,3,3,3,4),(-79.4909727263495,-78.4972990335714,-77.5036623369439,-76.5100256403164,
-75.5163889436889,-74.5227522470614,-73.5291155504339,-73.2077874191699),
 .UNSPECIFIED.);
#835=B_SPLINE_CURVE_WITH_KNOTS('',3,(#46666,#46667,#46668,#46669,#46670,
#46671,#46672,#46673,#46674,#46675,#46676,#46677,#46678,#46679,#46680,#46681,
#46682,#46683,#46684,#46685,#46686,#46687),.UNSPECIFIED.,.F.,.F.,(4,3,3,
3,3,3,3,4),(70.2250835898869,70.5482054605515,71.5418421571789,72.5354788538064,
73.5291155504339,74.5227522470614,75.5163889436889,76.5082688970665),
 .UNSPECIFIED.);
#836=B_SPLINE_CURVE_WITH_KNOTS('',3,(#46692,#46693,#46694,#46695,#46696,
#46697,#46698,#46699,#46700,#46701,#46702,#46703,#46704,#46705,#46706,#46707,
#46708,#46709,#46710,#46711,#46712,#46713),.UNSPECIFIED.,.F.,.F.,(4,3,3,
3,3,3,3,4),(-85.7741580335291,-85.4527559099638,-84.4591192133363,-83.4654825167088,
-82.4718458200813,-81.4782091234538,-80.4845724268263,-79.4909727263495),
 .UNSPECIFIED.);
#837=B_SPLINE_CURVE_WITH_KNOTS('',3,(#46714,#46715,#46716,#46717,#46718,
#46719,#46720,#46721,#46722,#46723,#46724,#46725,#46726,#46727,#46728,#46729,
#46730,#46731,#46732,#46733,#46734,#46735),.UNSPECIFIED.,.F.,.F.,(4,3,3,
3,3,3,3,4),(76.5082688970665,77.5036623369438,78.4972990335713,79.4909357301988,
80.4845724268263,81.4782091234538,82.4718458200813,82.7914542042461),
 .UNSPECIFIED.);
#838=B_SPLINE_CURVE_WITH_KNOTS('',3,(#46740,#46741,#46742,#46743,#46744,
#46745,#46746,#46747,#46748,#46749,#46750,#46751,#46752,#46753,#46754,#46755,
#46756,#46757,#46758,#46759,#46760,#46761),.UNSPECIFIED.,.F.,.F.,(4,3,3,
3,3,3,3,4),(-92.0573433407087,-91.4145760897287,-90.4209393931012,-89.4273026964737,
-88.4336659998462,-87.4400293032187,-86.4463926065912,-85.7741580335291),
 .UNSPECIFIED.);
#839=B_SPLINE_CURVE_WITH_KNOTS('',3,(#46762,#46763,#46764,#46765,#46766,
#46767,#46768,#46769,#46770,#46771,#46772,#46773,#46774,#46775,#46776,#46777,
#46778,#46779,#46780,#46781,#46782,#46783),.UNSPECIFIED.,.F.,.F.,(4,3,3,
3,3,3,3,4),(82.7914542042461,83.4654825167088,84.4591192133363,85.4527559099638,
86.4463926065912,87.4400293032187,88.4336659998462,89.0746395114257),
 .UNSPECIFIED.);
#840=B_SPLINE_CURVE_WITH_KNOTS('',3,(#46789,#46790,#46791,#46792,#46793),
 .UNSPECIFIED.,.F.,.F.,(4,1,4),(103.672557568463,104.023427014111,104.943135506477),
 .UNSPECIFIED.);
#841=B_SPLINE_CURVE_WITH_KNOTS('',3,(#46796,#46797,#46798,#46799),
 .UNSPECIFIED.,.F.,.F.,(4,4),(103.672557568463,103.703855626096),
 .UNSPECIFIED.);
#842=B_SPLINE_CURVE_WITH_KNOTS('',3,(#46804,#46805,#46806,#46807,#46808,
#46809,#46810,#46811,#46812,#46813),.UNSPECIFIED.,.F.,.F.,(4,1,1,1,1,1,
1,4),(97.3893722612836,98.0616068343457,99.0552435309732,100.048880227601,
101.042516924228,102.036153620856,103.029790317483,103.672557568463),
 .UNSPECIFIED.);
#843=B_SPLINE_CURVE_WITH_KNOTS('',3,(#46814,#46815,#46816,#46817,#46818,
#46819,#46820,#46821,#46822,#46823,#46824),.UNSPECIFIED.,.F.,.F.,(4,1,1,
1,1,1,1,1,4),(97.3893722612836,97.7420354463315,98.735672142959,99.7293088395865,
100.722945536214,101.716582232841,102.710218929469,103.207037277783,103.672557568463),
 .UNSPECIFIED.);
#844=B_SPLINE_CURVE_WITH_KNOTS('',3,(#46829,#46830,#46831,#46832,#46833,
#46834,#46835,#46836,#46837,#46838),.UNSPECIFIED.,.F.,.F.,(4,1,1,1,1,1,
1,4),(91.106186954104,92.0997866545808,93.0934233512083,94.0870600478358,
95.0806967444633,96.0743334410907,97.0679701377182,97.3893722612836),
 .UNSPECIFIED.);
#845=B_SPLINE_CURVE_WITH_KNOTS('',3,(#46839,#46840,#46841,#46842,#46843,
#46844,#46845,#46846,#46847,#46848),.UNSPECIFIED.,.F.,.F.,(4,1,1,1,1,1,
1,4),(91.106186954104,91.7802152665666,92.7738519631941,93.7674886598216,
94.761125356449,95.7547620530765,96.748398749704,97.3893722612836),
 .UNSPECIFIED.);
#846=B_SPLINE_CURVE_WITH_KNOTS('',3,(#46853,#46854,#46855,#46856,#46857,
#46858,#46859,#46860,#46861,#46862,#46863),.UNSPECIFIED.,.F.,.F.,(4,1,1,
1,1,1,1,1,4),(84.8230016469244,85.1443297781884,86.1379664748159,87.1316031714434,
88.1252398680709,89.1188765646984,90.1125132613258,91.1061499579533,91.106186954104),
 .UNSPECIFIED.);
#847=B_SPLINE_CURVE_WITH_KNOTS('',3,(#46864,#46865,#46866,#46867,#46868,
#46869,#46870,#46871,#46872,#46873,#46874),.UNSPECIFIED.,.F.,.F.,(4,1,1,
1,1,1,1,1,4),(84.8230016469244,84.8247583901742,85.8183950868017,86.8120317834291,
87.8056684800567,88.7993051766841,89.7929418733116,90.7865785699391,91.106186954104),
 .UNSPECIFIED.);
#848=B_SPLINE_CURVE_WITH_KNOTS('',3,(#46879,#46880,#46881,#46882,#46883,
#46884,#46885,#46886,#46887,#46888),.UNSPECIFIED.,.F.,.F.,(4,1,1,1,1,1,
1,4),(78.5398163397448,79.1825095984235,80.176146295051,81.1697829916785,
82.163419688306,83.1570563849334,84.1506930815609,84.8230016469244),
 .UNSPECIFIED.);
#849=B_SPLINE_CURVE_WITH_KNOTS('',3,(#46889,#46890,#46891,#46892,#46893,
#46894,#46895,#46896,#46897,#46898),.UNSPECIFIED.,.F.,.F.,(4,1,1,1,1,1,
1,4),(78.5398163397448,78.8629382104093,79.8565749070368,80.8502116036642,
81.8438483002917,82.8374849969192,83.8311216935467,84.8230016469244),
 .UNSPECIFIED.);
#850=B_SPLINE_CURVE_WITH_KNOTS('',3,(#46903,#46904,#46905,#46906,#46907,
#46908,#46909,#46910,#46911,#46912),.UNSPECIFIED.,.F.,.F.,(4,1,1,1,1,1,
1,4),(72.2566310325652,73.2206894186586,74.2143261152861,75.2079628119136,
76.201599508541,77.1952362051685,78.188872901796,78.5398163397448),
 .UNSPECIFIED.);
#851=B_SPLINE_CURVE_WITH_KNOTS('',3,(#46913,#46914,#46915,#46916,#46917,
#46918,#46919,#46920,#46921,#46922),.UNSPECIFIED.,.F.,.F.,(4,1,1,1,1,1,
1,4),(72.2566310325652,72.9011180306444,73.8947547272718,74.8883914238993,
75.8820281205268,76.8756648171543,77.8693015137818,78.5398163397448),
 .UNSPECIFIED.);
#852=B_SPLINE_CURVE_WITH_KNOTS('',3,(#46927,#46928,#46929,#46930,#46931,
#46932,#46933,#46934,#46935,#46936,#46937),.UNSPECIFIED.,.F.,.F.,(4,1,1,
1,1,1,1,1,4),(65.9734457253856,66.2652325422662,67.2588692388937,68.2525059355212,
69.2461426321486,70.2397793287761,71.2334160254036,72.2270527220311,72.2566310325652),
 .UNSPECIFIED.);
#853=B_SPLINE_CURVE_WITH_KNOTS('',3,(#46938,#46939,#46940,#46941,#46942,
#46943,#46944,#46945,#46946,#46947),.UNSPECIFIED.,.F.,.F.,(4,1,1,1,1,1,
1,4),(65.9734457253856,66.9392978508795,67.9329345475069,68.9265712441344,
69.9202079407619,70.9138446373894,71.9074813340169,72.2566310325652),
 .UNSPECIFIED.);
#854=B_SPLINE_CURVE_WITH_KNOTS('',3,(#46952,#46953,#46954,#46955,#46956,
#46957,#46958,#46959,#46960,#46961),.UNSPECIFIED.,.F.,.F.,(4,1,1,1,1,1,
1,4),(59.690260418206,60.3034123625013,61.2970490591288,62.2906857557562,
63.2843224523837,64.2779591490112,65.2715958456387,65.9734457253856),
 .UNSPECIFIED.);
#855=B_SPLINE_CURVE_WITH_KNOTS('',3,(#46962,#46963,#46964,#46965,#46966,
#46967,#46968,#46969,#46970,#46971,#46972),.UNSPECIFIED.,.F.,.F.,(4,1,1,
1,1,1,1,1,4),(59.690260418206,59.9838409744871,60.9774776711145,61.971114367742,
62.9647510643695,63.958387760997,64.9520244576245,65.945661154252,65.9734457253856),
 .UNSPECIFIED.);
#856=B_SPLINE_CURVE_WITH_KNOTS('',3,(#46977,#46978,#46979,#46980,#46981,
#46982,#46983,#46984,#46985,#46986),.UNSPECIFIED.,.F.,.F.,(4,1,1,1,1,1,
1,4),(53.4070751110265,54.3415921827364,55.3352288793638,56.3288655759913,
57.3225022726188,58.3161389692463,59.3097756658738,59.690260418206),
 .UNSPECIFIED.);
#857=B_SPLINE_CURVE_WITH_KNOTS('',3,(#46987,#46988,#46989,#46990,#46991,
#46992,#46993,#46994,#46995,#46996),.UNSPECIFIED.,.F.,.F.,(4,1,1,1,1,1,
1,4),(53.4070751110264,54.0220207947221,55.0156574913496,56.0092941879771,
57.0029308846046,57.9965675812321,58.9902042778596,59.690260418206),
 .UNSPECIFIED.);
#858=B_SPLINE_CURVE_WITH_KNOTS('',3,(#47001,#47002,#47003,#47004,#47005,
#47006,#47007,#47008,#47009,#47010,#47011),.UNSPECIFIED.,.F.,.F.,(4,1,1,
1,1,1,1,1,4),(47.1238898038469,47.386135306344,48.3797720029714,49.3734086995989,
50.3670453962264,51.3606820928539,52.3543187894814,53.3479554861089,53.4070751110265),
 .UNSPECIFIED.);
#859=B_SPLINE_CURVE_WITH_KNOTS('',3,(#47012,#47013,#47014,#47015,#47016,
#47017,#47018,#47019,#47020,#47021),.UNSPECIFIED.,.F.,.F.,(4,1,1,1,1,1,
1,4),(47.1238898038469,48.0602006149572,49.0538373115847,50.0474740082122,
51.0411107048397,52.0347474014672,53.0283840980947,53.4070751110264),
 .UNSPECIFIED.);
#860=B_SPLINE_CURVE_WITH_KNOTS('',3,(#47026,#47027,#47028,#47029,#47030,
#47031,#47032,#47033,#47034,#47035),.UNSPECIFIED.,.F.,.F.,(4,1,1,1,1,1,
1,4),(40.8407044966672,41.4243151265791,42.4179518232065,43.411588519834,
44.4052252164615,45.398861913089,46.3924986097165,47.1238898038469),
 .UNSPECIFIED.);
#861=B_SPLINE_CURVE_WITH_KNOTS('',3,(#47036,#47037,#47038,#47039,#47040,
#47041,#47042,#47043,#47044,#47045,#47046),.UNSPECIFIED.,.F.,.F.,(4,1,1,
1,1,1,1,1,4),(40.8407044966673,41.1047437385648,42.0983804351923,43.0920171318198,
44.0856538284473,45.0792905250748,46.0729272217023,47.0665639183297,47.1238898038469),
 .UNSPECIFIED.);
#862=B_SPLINE_CURVE_WITH_KNOTS('',3,(#47051,#47052,#47053,#47054,#47055,
#47056,#47057,#47058,#47059,#47060),.UNSPECIFIED.,.F.,.F.,(4,1,1,1,1,1,
1,4),(34.5575191894877,35.4624949468141,36.4561316434416,37.4497683400691,
38.4434050366966,39.4370417333241,40.4306784299516,40.8407044966672),
 .UNSPECIFIED.);
#863=B_SPLINE_CURVE_WITH_KNOTS('',3,(#47061,#47062,#47063,#47064,#47065,
#47066,#47067,#47068,#47069,#47070),.UNSPECIFIED.,.F.,.F.,(4,1,1,1,1,1,
1,4),(34.5575191894877,35.1429235587999,36.1365602554274,37.1301969520549,
38.1238336486824,39.1174703453099,40.1111070419373,40.8407044966673),
 .UNSPECIFIED.);
#864=B_SPLINE_CURVE_WITH_KNOTS('',3,(#47075,#47076,#47077,#47078,#47079,
#47080,#47081,#47082,#47083,#47084,#47085),.UNSPECIFIED.,.F.,.F.,(4,1,1,
1,1,1,1,1,4),(28.2743338823081,28.5070380704217,29.5006747670492,30.4943114636767,
31.4879481603042,32.4815848569317,33.4752215535592,34.4688582501867,34.5575191894877),
 .UNSPECIFIED.);
#865=B_SPLINE_CURVE_WITH_KNOTS('',3,(#47086,#47087,#47088,#47089,#47090,
#47091,#47092,#47093,#47094,#47095),.UNSPECIFIED.,.F.,.F.,(4,1,1,1,1,1,
1,4),(28.2743338823081,29.181103379035,30.1747400756625,31.16837677229,
32.1620134689175,33.155650165545,34.1492868621724,34.5575191894877),
 .UNSPECIFIED.);
#866=B_SPLINE_CURVE_WITH_KNOTS('',3,(#47100,#47101,#47102,#47103,#47104,
#47105,#47106,#47107,#47108,#47109),.UNSPECIFIED.,.F.,.F.,(4,1,1,1,1,1,
1,4),(21.9911485751285,22.5452178906568,23.5388545872843,24.5324912839118,
25.5261279805393,26.5197646771668,27.5134013737943,28.2743338823081),
 .UNSPECIFIED.);
#867=B_SPLINE_CURVE_WITH_KNOTS('',3,(#47110,#47111,#47112,#47113,#47114,
#47115,#47116,#47117,#47118,#47119,#47120),.UNSPECIFIED.,.F.,.F.,(4,1,1,
1,1,1,1,1,4),(21.9911485751285,22.2256465026426,23.2192831992701,24.2129198958976,
25.2065565925251,26.2001932891526,27.19382998578,28.1874666824075,28.2743338823081),
 .UNSPECIFIED.);
#868=B_SPLINE_CURVE_WITH_KNOTS('',3,(#47125,#47126,#47127,#47128,#47129,
#47130,#47131,#47132,#47133,#47134),.UNSPECIFIED.,.F.,.F.,(4,1,1,1,1,1,
1,4),(15.7079632679489,16.5833977108919,17.5770344075194,18.5706711041469,
19.5643078007744,20.5579444974019,21.5515811940293,21.9911485751285),
 .UNSPECIFIED.);
#869=B_SPLINE_CURVE_WITH_KNOTS('',3,(#47135,#47136,#47137,#47138,#47139,
#47140,#47141,#47142,#47143,#47144),.UNSPECIFIED.,.F.,.F.,(4,1,1,1,1,1,
1,4),(15.7079632679489,16.2638263228777,17.2574630195052,18.2510997161327,
19.2447364127602,20.2383731093876,21.2320098060151,21.9911485751285),
 .UNSPECIFIED.);
#870=B_SPLINE_CURVE_WITH_KNOTS('',3,(#47952,#47953,#47954,#47955,#47956,
#47957,#47958,#47959,#47960,#47961,#47962,#47963,#47964,#47965,#47966,#47967,
#47968,#47969,#47970,#47971,#47972,#47973,#47974,#47975,#47976,#47977,#47978,
#47979,#47980,#47981,#47982,#47983,#47984,#47985,#47986,#47987,#47988,#47989,
#47990,#47991,#47992,#47993,#47994,#47995,#47996,#47997,#47998,#47999,#48000,
#48001,#48002,#48003,#48004,#48005,#48006,#48007,#48008,#48009,#48010,#48011,
#48012,#48013,#48014,#48015),.UNSPECIFIED.,.F.,.F.,(4,3,3,3,3,3,3,3,3,3,
3,3,3,3,3,3,3,3,3,3,3,4),(-0.741270768406293,-0.712255887547373,-0.665684585950267,
-0.644578145540201,-0.627409884287908,-0.56289444703525,-0.543149871110002,
-0.525346816277411,-0.462778575991627,-0.422541646340016,-0.403602109472732,
-0.388134731867962,-0.339685474770525,-0.287921025014436,-0.267367512869476,
-0.250461281201999,-0.191574752108606,-0.165649592692258,-0.130279761088628,
-0.116485368772831,-0.0582426843864153,0.),.UNSPECIFIED.);
#871=B_SPLINE_CURVE_WITH_KNOTS('',3,(#48016,#48017,#48018,#48019,#48020,
#48021,#48022,#48023,#48024,#48025,#48026,#48027,#48028,#48029,#48030,#48031),
 .UNSPECIFIED.,.F.,.F.,(4,3,3,3,3,4),(89.0746395114257,89.4273026964737,
90.4209393931012,91.4145760897287,92.4082127863561,93.3279212787228),
 .UNSPECIFIED.);
#872=B_SPLINE_CURVE_WITH_KNOTS('',3,(#48033,#48034,#48035,#48036,#48037,
#48038,#48039,#48040,#48041,#48042,#48043,#48044,#48045,#48046,#48047,#48048,
#48049,#48050,#48051,#48052,#48053,#48054,#48055,#48056,#48057,#48058,#48059,
#48060,#48061,#48062,#48063,#48064,#48065,#48066,#48067,#48068,#48069,#48070,
#48071,#48072,#48073,#48074,#48075,#48076,#48077,#48078,#48079,#48080,#48081,
#48082,#48083,#48084,#48085,#48086,#48087,#48088,#48089,#48090,#48091,#48092,
#48093,#48094,#48095,#48096),.UNSPECIFIED.,.F.,.F.,(4,3,3,3,3,3,3,3,3,3,
3,3,3,3,3,3,3,3,3,3,3,4),(-0.744397949170265,-0.720232764262911,-0.673202521468055,
-0.646203568187049,-0.596939292083825,-0.573499405051569,-0.555762434684145,
-0.495454099387841,-0.456502934283493,-0.439348901583241,-0.424325906339616,
-0.376932525681518,-0.330843929367177,-0.304626791409719,-0.285107413231915,
-0.222343876864638,-0.192578140424153,-0.156226789527131,-0.140024719995705,
-0.0753705999558412,-0.0106626303314335,0.),.UNSPECIFIED.);
#873=B_SPLINE_CURVE_WITH_KNOTS('',3,(#48097,#48098,#48099,#48100,#48101,
#48102,#48103,#48104,#48105),.UNSPECIFIED.,.F.,.F.,(4,1,1,1,1,1,4),(10.3759343473736,
11.2956428397403,12.2892795363678,13.2829162329952,14.2765529296227,15.2701896262502,
15.7079632679489),.UNSPECIFIED.);
#874=B_SPLINE_CURVE_WITH_KNOTS('',3,(#48111,#48112,#48113,#48114,#48115,
#48116,#48117,#48118,#48119,#48120,#48121,#48122,#48123,#48124,#48125,#48126,
#48127,#48128,#48129,#48130,#48131,#48132,#48133,#48134,#48135,#48136,#48137,
#48138,#48139,#48140,#48141,#48142,#48143,#48144,#48145,#48146,#48147,#48148,
#48149,#48150,#48151,#48152,#48153,#48154,#48155,#48156,#48157,#48158,#48159,
#48160,#48161,#48162,#48163,#48164,#48165,#48166,#48167,#48168,#48169,#48170,
#48171,#48172,#48173,#48174),.UNSPECIFIED.,.F.,.F.,(4,3,3,3,3,3,3,3,3,3,
3,3,3,3,3,3,3,3,3,3,3,4),(-0.741270768406662,-0.712255887547674,-0.665684585950538,
-0.644578143487901,-0.627409881579087,-0.562894446898948,-0.543149865542399,
-0.525346815316762,-0.462778578250359,-0.4225416506717,-0.403602129361835,
-0.388134740123997,-0.339685474770589,-0.287920989652608,-0.267367466812484,
-0.250461299706187,-0.191574764229376,-0.165649592692285,-0.130279760406768,
-0.116485367671245,-0.0582426838356225,0.),.UNSPECIFIED.);
#875=B_SPLINE_CURVE_WITH_KNOTS('',3,(#48177,#48178,#48179,#48180,#48181,
#48182,#48183,#48184,#48185),.UNSPECIFIED.,.F.,.F.,(4,1,1,1,1,1,4),(11.6152142277545,
12.1120325760682,12.608850924382,13.6024876210095,14.5961243176369,15.5897610142644,
15.7079632679489),.UNSPECIFIED.);
#876=B_SPLINE_CURVE_WITH_KNOTS('',3,(#48591,#48592,#48593,#48594,#48595,
#48596,#48597,#48598,#48599,#48600,#48601,#48602,#48603,#48604,#48605,#48606,
#48607,#48608,#48609,#48610,#48611,#48612,#48613,#48614,#48615,#48616,#48617,
#48618,#48619,#48620,#48621,#48622,#48623,#48624,#48625,#48626,#48627,#48628,
#48629,#48630,#48631,#48632,#48633,#48634,#48635,#48636,#48637,#48638,#48639,
#48640,#48641,#48642,#48643,#48644,#48645,#48646,#48647,#48648,#48649,#48650,
#48651,#48652,#48653,#48654),.UNSPECIFIED.,.F.,.F.,(4,3,3,3,3,3,3,3,3,3,
3,3,3,3,3,3,3,3,3,3,3,4),(-0.744397949170718,-0.720232764263358,-0.673202521370767,
-0.646203568277415,-0.596939266463238,-0.573498931627384,-0.555762400888746,
-0.495454066743922,-0.456502918787901,-0.439348839381182,-0.424325811011317,
-0.376932525681586,-0.330843929367237,-0.304626788677627,-0.285107412643743,
-0.222343877199312,-0.19257814042419,-0.156226788834009,-0.140024719746733,
-0.0753705894557632,-0.0106626208978399,0.),.UNSPECIFIED.);
#877=B_SPLINE_CURVE_WITH_KNOTS('',3,(#48655,#48656,#48657,#48658,#48659,
#48660,#48661,#48662,#48663,#48664,#48665,#48666,#48667,#48668,#48669,#48670),
 .UNSPECIFIED.,.F.,.F.,(4,3,3,3,3,4),(-95.3891228762386,-94.8923045279249,
-94.3954861796111,-93.4018494829836,-92.4082127863561,-92.0573433407087),
 .UNSPECIFIED.);
#1456=B_SPLINE_SURFACE_WITH_KNOTS('',3,3,((#47547,#47548,#47549,#47550,
#47551,#47552,#47553,#47554,#47555,#47556,#47557,#47558,#47559,#47560,#47561,
#47562,#47563,#47564,#47565,#47566,#47567,#47568,#47569,#47570,#47571,#47572,
#47573,#47574,#47575,#47576,#47577,#47578,#47579,#47580,#47581,#47582,#47583,
#47584,#47585,#47586,#47587,#47588,#47589,#47590,#47591,#47592,#47593,#47594,
#47595,#47596,#47597,#47598,#47599,#47600,#47601,#47602,#47603,#47604,#47605,
#47606,#47607,#47608,#47609,#47610,#47611,#47612,#47613,#47614,#47615,#47616,
#47617,#47618,#47619,#47620,#47621,#47622,#47623,#47624,#47625,#47626,#47627,
#47628,#47629,#47630,#47631,#47632,#47633,#47634,#47635,#47636,#47637,#47638,
#47639,#47640,#47641,#47642,#47643,#47644,#47645,#47646,#47647),(#47648,
#47649,#47650,#47651,#47652,#47653,#47654,#47655,#47656,#47657,#47658,#47659,
#47660,#47661,#47662,#47663,#47664,#47665,#47666,#47667,#47668,#47669,#47670,
#47671,#47672,#47673,#47674,#47675,#47676,#47677,#47678,#47679,#47680,#47681,
#47682,#47683,#47684,#47685,#47686,#47687,#47688,#47689,#47690,#47691,#47692,
#47693,#47694,#47695,#47696,#47697,#47698,#47699,#47700,#47701,#47702,#47703,
#47704,#47705,#47706,#47707,#47708,#47709,#47710,#47711,#47712,#47713,#47714,
#47715,#47716,#47717,#47718,#47719,#47720,#47721,#47722,#47723,#47724,#47725,
#47726,#47727,#47728,#47729,#47730,#47731,#47732,#47733,#47734,#47735,#47736,
#47737,#47738,#47739,#47740,#47741,#47742,#47743,#47744,#47745,#47746,#47747,
#47748),(#47749,#47750,#47751,#47752,#47753,#47754,#47755,#47756,#47757,
#47758,#47759,#47760,#47761,#47762,#47763,#47764,#47765,#47766,#47767,#47768,
#47769,#47770,#47771,#47772,#47773,#47774,#47775,#47776,#47777,#47778,#47779,
#47780,#47781,#47782,#47783,#47784,#47785,#47786,#47787,#47788,#47789,#47790,
#47791,#47792,#47793,#47794,#47795,#47796,#47797,#47798,#47799,#47800,#47801,
#47802,#47803,#47804,#47805,#47806,#47807,#47808,#47809,#47810,#47811,#47812,
#47813,#47814,#47815,#47816,#47817,#47818,#47819,#47820,#47821,#47822,#47823,
#47824,#47825,#47826,#47827,#47828,#47829,#47830,#47831,#47832,#47833,#47834,
#47835,#47836,#47837,#47838,#47839,#47840,#47841,#47842,#47843,#47844,#47845,
#47846,#47847,#47848,#47849),(#47850,#47851,#47852,#47853,#47854,#47855,
#47856,#47857,#47858,#47859,#47860,#47861,#47862,#47863,#47864,#47865,#47866,
#47867,#47868,#47869,#47870,#47871,#47872,#47873,#47874,#47875,#47876,#47877,
#47878,#47879,#47880,#47881,#47882,#47883,#47884,#47885,#47886,#47887,#47888,
#47889,#47890,#47891,#47892,#47893,#47894,#47895,#47896,#47897,#47898,#47899,
#47900,#47901,#47902,#47903,#47904,#47905,#47906,#47907,#47908,#47909,#47910,
#47911,#47912,#47913,#47914,#47915,#47916,#47917,#47918,#47919,#47920,#47921,
#47922,#47923,#47924,#47925,#47926,#47927,#47928,#47929,#47930,#47931,#47932,
#47933,#47934,#47935,#47936,#47937,#47938,#47939,#47940,#47941,#47942,#47943,
#47944,#47945,#47946,#47947,#47948,#47949,#47950)),.UNSPECIFIED.,.F.,.F.,
 .F.,(4,4),(4,1,1,1,1,1,1,1,1,1,1,1,1,1,1,1,1,1,1,1,1,1,1,1,1,1,1,1,1,1,
1,1,1,1,1,1,1,1,1,1,1,1,1,1,1,1,1,1,1,1,1,1,1,1,1,1,1,1,1,1,1,1,1,1,1,1,
1,1,1,1,1,1,1,1,1,1,1,1,1,1,1,1,1,1,1,1,1,1,1,1,1,1,1,1,1,1,1,1,4),(0.,
0.0820126057383864),(8.31473274985782,8.81155109817156,9.3083694464853,
10.3020061431128,11.2956428397403,12.2892795363678,13.2829162329952,14.2765529296227,
15.2701896262502,16.2638263228777,17.2574630195052,18.2510997161327,19.2447364127602,
20.2383731093876,21.2320098060151,22.2256465026426,23.2192831992701,24.2129198958976,
25.2065565925251,26.2001932891526,27.19382998578,28.1874666824075,29.181103379035,
30.1747400756625,31.16837677229,32.1620134689175,33.155650165545,34.1492868621724,
35.1429235587999,36.1365602554274,37.1301969520549,38.1238336486824,39.1174703453099,
40.1111070419373,41.1047437385648,42.0983804351923,43.0920171318198,44.0856538284473,
45.0792905250748,46.0729272217023,47.0665639183297,48.0602006149572,49.0538373115847,
50.0474740082122,51.0411107048397,52.0347474014672,53.0283840980947,54.0220207947221,
55.0156574913496,56.0092941879771,57.0029308846046,57.9965675812321,58.9902042778596,
59.9838409744871,60.9774776711145,61.971114367742,62.9647510643695,63.958387760997,
64.9520244576245,65.945661154252,66.9392978508795,67.9329345475069,68.9265712441344,
69.9202079407619,70.9138446373894,71.9074813340169,72.9011180306444,73.8947547272718,
74.8883914238993,75.8820281205268,76.8756648171543,77.8693015137818,78.8629382104093,
79.8565749070368,80.8502116036642,81.8438483002917,82.8374849969192,83.8311216935467,
84.8247583901742,85.8183950868017,86.8120317834291,87.8056684800567,88.7993051766841,
89.7929418733116,90.7865785699391,91.7802152665666,92.7738519631941,93.7674886598216,
94.761125356449,95.7547620530765,96.748398749704,97.7420354463315,98.735672142959,
99.7293088395865,100.722945536214,101.716582232841,102.710218929469,103.207037277783,
103.703855626096),.UNSPECIFIED.);
#1457=B_SPLINE_SURFACE_WITH_KNOTS('',3,3,((#48186,#48187,#48188,#48189,
#48190,#48191,#48192,#48193,#48194,#48195,#48196,#48197,#48198,#48199,#48200,
#48201,#48202,#48203,#48204,#48205,#48206,#48207,#48208,#48209,#48210,#48211,
#48212,#48213,#48214,#48215,#48216,#48217,#48218,#48219,#48220,#48221,#48222,
#48223,#48224,#48225,#48226,#48227,#48228,#48229,#48230,#48231,#48232,#48233,
#48234,#48235,#48236,#48237,#48238,#48239,#48240,#48241,#48242,#48243,#48244,
#48245,#48246,#48247,#48248,#48249,#48250,#48251,#48252,#48253,#48254,#48255,
#48256,#48257,#48258,#48259,#48260,#48261,#48262,#48263,#48264,#48265,#48266,
#48267,#48268,#48269,#48270,#48271,#48272,#48273,#48274,#48275,#48276,#48277,
#48278,#48279,#48280,#48281,#48282,#48283,#48284,#48285,#48286),(#48287,
#48288,#48289,#48290,#48291,#48292,#48293,#48294,#48295,#48296,#48297,#48298,
#48299,#48300,#48301,#48302,#48303,#48304,#48305,#48306,#48307,#48308,#48309,
#48310,#48311,#48312,#48313,#48314,#48315,#48316,#48317,#48318,#48319,#48320,
#48321,#48322,#48323,#48324,#48325,#48326,#48327,#48328,#48329,#48330,#48331,
#48332,#48333,#48334,#48335,#48336,#48337,#48338,#48339,#48340,#48341,#48342,
#48343,#48344,#48345,#48346,#48347,#48348,#48349,#48350,#48351,#48352,#48353,
#48354,#48355,#48356,#48357,#48358,#48359,#48360,#48361,#48362,#48363,#48364,
#48365,#48366,#48367,#48368,#48369,#48370,#48371,#48372,#48373,#48374,#48375,
#48376,#48377,#48378,#48379,#48380,#48381,#48382,#48383,#48384,#48385,#48386,
#48387),(#48388,#48389,#48390,#48391,#48392,#48393,#48394,#48395,#48396,
#48397,#48398,#48399,#48400,#48401,#48402,#48403,#48404,#48405,#48406,#48407,
#48408,#48409,#48410,#48411,#48412,#48413,#48414,#48415,#48416,#48417,#48418,
#48419,#48420,#48421,#48422,#48423,#48424,#48425,#48426,#48427,#48428,#48429,
#48430,#48431,#48432,#48433,#48434,#48435,#48436,#48437,#48438,#48439,#48440,
#48441,#48442,#48443,#48444,#48445,#48446,#48447,#48448,#48449,#48450,#48451,
#48452,#48453,#48454,#48455,#48456,#48457,#48458,#48459,#48460,#48461,#48462,
#48463,#48464,#48465,#48466,#48467,#48468,#48469,#48470,#48471,#48472,#48473,
#48474,#48475,#48476,#48477,#48478,#48479,#48480,#48481,#48482,#48483,#48484,
#48485,#48486,#48487,#48488),(#48489,#48490,#48491,#48492,#48493,#48494,
#48495,#48496,#48497,#48498,#48499,#48500,#48501,#48502,#48503,#48504,#48505,
#48506,#48507,#48508,#48509,#48510,#48511,#48512,#48513,#48514,#48515,#48516,
#48517,#48518,#48519,#48520,#48521,#48522,#48523,#48524,#48525,#48526,#48527,
#48528,#48529,#48530,#48531,#48532,#48533,#48534,#48535,#48536,#48537,#48538,
#48539,#48540,#48541,#48542,#48543,#48544,#48545,#48546,#48547,#48548,#48549,
#48550,#48551,#48552,#48553,#48554,#48555,#48556,#48557,#48558,#48559,#48560,
#48561,#48562,#48563,#48564,#48565,#48566,#48567,#48568,#48569,#48570,#48571,
#48572,#48573,#48574,#48575,#48576,#48577,#48578,#48579,#48580,#48581,#48582,
#48583,#48584,#48585,#48586,#48587,#48588,#48589)),.UNSPECIFIED.,.F.,.F.,
 .F.,(4,4),(4,1,1,1,1,1,1,1,1,1,1,1,1,1,1,1,1,1,1,1,1,1,1,1,1,1,1,1,1,1,
1,1,1,1,1,1,1,1,1,1,1,1,1,1,1,1,1,1,1,1,1,1,1,1,1,1,1,1,1,1,1,1,1,1,1,1,
1,1,1,1,1,1,1,1,1,1,1,1,1,1,1,1,1,1,1,1,1,1,1,1,1,1,1,1,1,1,1,1,4),(0.,
0.0820126057383864),(11.6152142277545,12.1120325760682,12.608850924382,
13.6024876210095,14.5961243176369,15.5897610142644,16.5833977108919,17.5770344075194,
18.5706711041469,19.5643078007744,20.5579444974019,21.5515811940293,22.5452178906568,
23.5388545872843,24.5324912839118,25.5261279805393,26.5197646771668,27.5134013737943,
28.5070380704217,29.5006747670492,30.4943114636767,31.4879481603042,32.4815848569317,
33.4752215535592,34.4688582501867,35.4624949468141,36.4561316434416,37.4497683400691,
38.4434050366966,39.4370417333241,40.4306784299516,41.4243151265791,42.4179518232065,
43.411588519834,44.4052252164615,45.398861913089,46.3924986097165,47.386135306344,
48.3797720029714,49.3734086995989,50.3670453962264,51.3606820928539,52.3543187894814,
53.3479554861089,54.3415921827364,55.3352288793638,56.3288655759913,57.3225022726188,
58.3161389692463,59.3097756658738,60.3034123625013,61.2970490591288,62.2906857557562,
63.2843224523837,64.2779591490112,65.2715958456387,66.2652325422662,67.2588692388937,
68.2525059355212,69.2461426321486,70.2397793287761,71.2334160254036,72.2270527220311,
73.2206894186586,74.2143261152861,75.2079628119136,76.201599508541,77.1952362051685,
78.188872901796,79.1825095984235,80.176146295051,81.1697829916785,82.163419688306,
83.1570563849334,84.1506930815609,85.1443297781884,86.1379664748159,87.1316031714434,
88.1252398680709,89.1188765646984,90.1125132613258,91.1061499579533,92.0997866545808,
93.0934233512083,94.0870600478358,95.0806967444633,96.0743334410907,97.0679701377182,
98.0616068343457,99.0552435309732,100.048880227601,101.042516924228,102.036153620856,
103.029790317483,104.023427014111,105.017063710738,106.010700407366,106.507518755679,
107.004337103993),.UNSPECIFIED.);
#1628=CYLINDRICAL_SURFACE('',#29737,0.3933);
#1629=CYLINDRICAL_SURFACE('',#29739,0.3933);
#1630=CYLINDRICAL_SURFACE('',#29740,0.3933);
#1631=CYLINDRICAL_SURFACE('',#29741,0.3933);
#1632=CYLINDRICAL_SURFACE('',#29742,0.3933);
#1633=CYLINDRICAL_SURFACE('',#29743,0.3933);
#1634=CYLINDRICAL_SURFACE('',#29744,0.3933);
#1635=CYLINDRICAL_SURFACE('',#29745,0.3933);
#1636=CYLINDRICAL_SURFACE('',#29746,0.3933);
#1637=CYLINDRICAL_SURFACE('',#29747,0.3933);
#1638=CYLINDRICAL_SURFACE('',#29748,0.3933);
#1639=CYLINDRICAL_SURFACE('',#29749,0.3933);
#1640=CYLINDRICAL_SURFACE('',#29750,0.3933);
#1641=CYLINDRICAL_SURFACE('',#29751,0.3933);
#1642=CYLINDRICAL_SURFACE('',#29752,0.3933);
#1643=CYLINDRICAL_SURFACE('',#29753,0.322275);
#1644=CYLINDRICAL_SURFACE('',#29755,0.322275);
#1645=CYLINDRICAL_SURFACE('',#29756,0.322275);
#1646=CYLINDRICAL_SURFACE('',#29757,0.322275);
#1647=CYLINDRICAL_SURFACE('',#29758,0.322275);
#1648=CYLINDRICAL_SURFACE('',#29759,0.322275);
#1649=CYLINDRICAL_SURFACE('',#29760,0.322275);
#1650=CYLINDRICAL_SURFACE('',#29761,0.322275);
#1651=CYLINDRICAL_SURFACE('',#29762,0.322275);
#1652=CYLINDRICAL_SURFACE('',#29763,0.322275);
#1653=CYLINDRICAL_SURFACE('',#29764,0.322275);
#1654=CYLINDRICAL_SURFACE('',#29765,0.322275);
#1655=CYLINDRICAL_SURFACE('',#29766,0.322275);
#1656=CYLINDRICAL_SURFACE('',#29767,0.322275);
#1657=CYLINDRICAL_SURFACE('',#29768,0.322275);
#1658=CYLINDRICAL_SURFACE('',#29842,1.1);
#1659=CYLINDRICAL_SURFACE('',#29866,0.322275);
#1660=CYLINDRICAL_SURFACE('',#29870,0.3933);
#1930=FACE_BOUND('',#5494,.T.);
#2400=CIRCLE('',#29738,0.3933);
#2401=CIRCLE('',#29754,0.322275);
#2402=CIRCLE('',#29771,1.1);
#2403=CIRCLE('',#29775,1.1);
#2404=CIRCLE('',#29779,1.1);
#2405=CIRCLE('',#29783,1.1);
#2406=CIRCLE('',#29787,1.1);
#2407=CIRCLE('',#29791,1.1);
#2408=CIRCLE('',#29795,1.1);
#2409=CIRCLE('',#29799,1.1);
#2410=CIRCLE('',#29803,1.1);
#2411=CIRCLE('',#29807,1.1);
#2412=CIRCLE('',#29811,1.1);
#2413=CIRCLE('',#29815,1.1);
#2414=CIRCLE('',#29819,1.1);
#2415=CIRCLE('',#29823,1.1);
#2416=CIRCLE('',#29824,1.1);
#2417=CIRCLE('',#29828,1.1);
#2418=CIRCLE('',#29832,1.1);
#2419=CIRCLE('',#29836,1.1);
#2420=CIRCLE('',#29840,1.1);
#2421=CIRCLE('',#29843,1.1);
#2422=CIRCLE('',#29844,1.1);
#2423=CIRCLE('',#29845,1.1);
#2424=CIRCLE('',#29846,1.1);
#2425=CIRCLE('',#29847,1.1);
#2426=CIRCLE('',#29848,1.1);
#2427=CIRCLE('',#29849,1.1);
#2428=CIRCLE('',#29850,1.1);
#2429=CIRCLE('',#29851,1.1);
#2430=CIRCLE('',#29852,1.1);
#2431=CIRCLE('',#29853,1.1);
#2432=CIRCLE('',#29854,1.1);
#2433=CIRCLE('',#29855,1.1);
#2434=CIRCLE('',#29856,1.1);
#2435=CIRCLE('',#29857,1.1);
#2436=CIRCLE('',#29858,1.1);
#2437=CIRCLE('',#29859,1.1);
#2438=CIRCLE('',#29860,1.1);
#2439=CIRCLE('',#29861,1.1);
#2440=CIRCLE('',#29863,0.3933);
#2441=CIRCLE('',#29864,0.3933);
#2442=CIRCLE('',#29865,0.322275);
#2443=CIRCLE('',#29868,0.35);
#2444=CIRCLE('',#29871,0.3933);
#2445=CIRCLE('',#29873,0.9);
#2446=CIRCLE('',#29876,1.);
#2856=CONICAL_SURFACE('',#29869,0.375,0.785398163397448);
#2857=CONICAL_SURFACE('',#29874,1.,0.785398163397445);
#2858=CONICAL_SURFACE('',#29875,1.05,0.463647609000806);
#3765=FACE_OUTER_BOUND('',#5401,.T.);
#3766=FACE_OUTER_BOUND('',#5402,.T.);
#3767=FACE_OUTER_BOUND('',#5403,.T.);
#3768=FACE_OUTER_BOUND('',#5404,.T.);
#3769=FACE_OUTER_BOUND('',#5405,.T.);
#3770=FACE_OUTER_BOUND('',#5406,.T.);
#3771=FACE_OUTER_BOUND('',#5407,.T.);
#3772=FACE_OUTER_BOUND('',#5408,.T.);
#3773=FACE_OUTER_BOUND('',#5409,.T.);
#3774=FACE_OUTER_BOUND('',#5410,.T.);
#3775=FACE_OUTER_BOUND('',#5411,.T.);
#3776=FACE_OUTER_BOUND('',#5412,.T.);
#3777=FACE_OUTER_BOUND('',#5413,.T.);
#3778=FACE_OUTER_BOUND('',#5414,.T.);
#3779=FACE_OUTER_BOUND('',#5415,.T.);
#3780=FACE_OUTER_BOUND('',#5416,.T.);
#3781=FACE_OUTER_BOUND('',#5417,.T.);
#3782=FACE_OUTER_BOUND('',#5418,.T.);
#3783=FACE_OUTER_BOUND('',#5419,.T.);
#3784=FACE_OUTER_BOUND('',#5420,.T.);
#3785=FACE_OUTER_BOUND('',#5421,.T.);
#3786=FACE_OUTER_BOUND('',#5422,.T.);
#3787=FACE_OUTER_BOUND('',#5423,.T.);
#3788=FACE_OUTER_BOUND('',#5424,.T.);
#3789=FACE_OUTER_BOUND('',#5425,.T.);
#3790=FACE_OUTER_BOUND('',#5426,.T.);
#3791=FACE_OUTER_BOUND('',#5427,.T.);
#3792=FACE_OUTER_BOUND('',#5428,.T.);
#3793=FACE_OUTER_BOUND('',#5429,.T.);
#3794=FACE_OUTER_BOUND('',#5430,.T.);
#3795=FACE_OUTER_BOUND('',#5431,.T.);
#3796=FACE_OUTER_BOUND('',#5432,.T.);
#3797=FACE_OUTER_BOUND('',#5433,.T.);
#3798=FACE_OUTER_BOUND('',#5434,.T.);
#3799=FACE_OUTER_BOUND('',#5435,.T.);
#3800=FACE_OUTER_BOUND('',#5436,.T.);
#3801=FACE_OUTER_BOUND('',#5437,.T.);
#3802=FACE_OUTER_BOUND('',#5438,.T.);
#3803=FACE_OUTER_BOUND('',#5439,.T.);
#3804=FACE_OUTER_BOUND('',#5440,.T.);
#3805=FACE_OUTER_BOUND('',#5441,.T.);
#3806=FACE_OUTER_BOUND('',#5442,.T.);
#3807=FACE_OUTER_BOUND('',#5443,.T.);
#3808=FACE_OUTER_BOUND('',#5444,.T.);
#3809=FACE_OUTER_BOUND('',#5445,.T.);
#3810=FACE_OUTER_BOUND('',#5446,.T.);
#3811=FACE_OUTER_BOUND('',#5447,.T.);
#3812=FACE_OUTER_BOUND('',#5448,.T.);
#3813=FACE_OUTER_BOUND('',#5449,.T.);
#3814=FACE_OUTER_BOUND('',#5450,.T.);
#3815=FACE_OUTER_BOUND('',#5451,.T.);
#3816=FACE_OUTER_BOUND('',#5452,.T.);
#3817=FACE_OUTER_BOUND('',#5453,.T.);
#3818=FACE_OUTER_BOUND('',#5454,.T.);
#3819=FACE_OUTER_BOUND('',#5455,.T.);
#3820=FACE_OUTER_BOUND('',#5456,.T.);
#3821=FACE_OUTER_BOUND('',#5457,.T.);
#3822=FACE_OUTER_BOUND('',#5458,.T.);
#3823=FACE_OUTER_BOUND('',#5459,.T.);
#3824=FACE_OUTER_BOUND('',#5460,.T.);
#3825=FACE_OUTER_BOUND('',#5461,.T.);
#3826=FACE_OUTER_BOUND('',#5462,.T.);
#3827=FACE_OUTER_BOUND('',#5463,.T.);
#3828=FACE_OUTER_BOUND('',#5464,.T.);
#3829=FACE_OUTER_BOUND('',#5465,.T.);
#3830=FACE_OUTER_BOUND('',#5466,.T.);
#3831=FACE_OUTER_BOUND('',#5467,.T.);
#3832=FACE_OUTER_BOUND('',#5468,.T.);
#3833=FACE_OUTER_BOUND('',#5469,.T.);
#3834=FACE_OUTER_BOUND('',#5470,.T.);
#3835=FACE_OUTER_BOUND('',#5471,.T.);
#3836=FACE_OUTER_BOUND('',#5472,.T.);
#3837=FACE_OUTER_BOUND('',#5473,.T.);
#3838=FACE_OUTER_BOUND('',#5474,.T.);
#3839=FACE_OUTER_BOUND('',#5475,.T.);
#3840=FACE_OUTER_BOUND('',#5476,.T.);
#3841=FACE_OUTER_BOUND('',#5477,.T.);
#3842=FACE_OUTER_BOUND('',#5478,.T.);
#3843=FACE_OUTER_BOUND('',#5479,.T.);
#3844=FACE_OUTER_BOUND('',#5480,.T.);
#3845=FACE_OUTER_BOUND('',#5481,.T.);
#3846=FACE_OUTER_BOUND('',#5482,.T.);
#3847=FACE_OUTER_BOUND('',#5483,.T.);
#3848=FACE_OUTER_BOUND('',#5484,.T.);
#3849=FACE_OUTER_BOUND('',#5485,.T.);
#3850=FACE_OUTER_BOUND('',#5486,.T.);
#3851=FACE_OUTER_BOUND('',#5487,.T.);
#3852=FACE_OUTER_BOUND('',#5488,.T.);
#3853=FACE_OUTER_BOUND('',#5489,.T.);
#3854=FACE_OUTER_BOUND('',#5490,.T.);
#3855=FACE_OUTER_BOUND('',#5491,.T.);
#3856=FACE_OUTER_BOUND('',#5492,.T.);
#3857=FACE_OUTER_BOUND('',#5493,.T.);
#3858=FACE_OUTER_BOUND('',#5495,.T.);
#3859=FACE_OUTER_BOUND('',#5496,.T.);
#3860=FACE_OUTER_BOUND('',#5497,.T.);
#5401=EDGE_LOOP('',(#22033,#22034,#22035,#22036));
#5402=EDGE_LOOP('',(#22037,#22038,#22039,#22040));
#5403=EDGE_LOOP('',(#22041,#22042,#22043,#22044));
#5404=EDGE_LOOP('',(#22045,#22046,#22047,#22048));
#5405=EDGE_LOOP('',(#22049,#22050,#22051,#22052));
#5406=EDGE_LOOP('',(#22053,#22054,#22055,#22056));
#5407=EDGE_LOOP('',(#22057,#22058,#22059,#22060));
#5408=EDGE_LOOP('',(#22061,#22062,#22063,#22064));
#5409=EDGE_LOOP('',(#22065,#22066,#22067,#22068));
#5410=EDGE_LOOP('',(#22069,#22070,#22071,#22072));
#5411=EDGE_LOOP('',(#22073,#22074,#22075,#22076));
#5412=EDGE_LOOP('',(#22077,#22078,#22079,#22080));
#5413=EDGE_LOOP('',(#22081,#22082,#22083,#22084));
#5414=EDGE_LOOP('',(#22085,#22086,#22087,#22088));
#5415=EDGE_LOOP('',(#22089,#22090,#22091,#22092));
#5416=EDGE_LOOP('',(#22093,#22094,#22095,#22096));
#5417=EDGE_LOOP('',(#22097,#22098,#22099,#22100));
#5418=EDGE_LOOP('',(#22101,#22102,#22103,#22104));
#5419=EDGE_LOOP('',(#22105,#22106,#22107,#22108));
#5420=EDGE_LOOP('',(#22109,#22110,#22111,#22112));
#5421=EDGE_LOOP('',(#22113,#22114,#22115,#22116));
#5422=EDGE_LOOP('',(#22117,#22118,#22119,#22120));
#5423=EDGE_LOOP('',(#22121,#22122,#22123,#22124));
#5424=EDGE_LOOP('',(#22125,#22126,#22127,#22128));
#5425=EDGE_LOOP('',(#22129,#22130,#22131,#22132));
#5426=EDGE_LOOP('',(#22133,#22134,#22135,#22136));
#5427=EDGE_LOOP('',(#22137,#22138,#22139,#22140));
#5428=EDGE_LOOP('',(#22141,#22142,#22143,#22144));
#5429=EDGE_LOOP('',(#22145,#22146,#22147,#22148));
#5430=EDGE_LOOP('',(#22149,#22150,#22151,#22152));
#5431=EDGE_LOOP('',(#22153,#22154,#22155,#22156));
#5432=EDGE_LOOP('',(#22157,#22158,#22159));
#5433=EDGE_LOOP('',(#22160,#22161,#22162,#22163));
#5434=EDGE_LOOP('',(#22164,#22165,#22166,#22167));
#5435=EDGE_LOOP('',(#22168,#22169,#22170));
#5436=EDGE_LOOP('',(#22171,#22172,#22173,#22174));
#5437=EDGE_LOOP('',(#22175,#22176,#22177,#22178));
#5438=EDGE_LOOP('',(#22179,#22180,#22181));
#5439=EDGE_LOOP('',(#22182,#22183,#22184,#22185));
#5440=EDGE_LOOP('',(#22186,#22187,#22188,#22189));
#5441=EDGE_LOOP('',(#22190,#22191,#22192));
#5442=EDGE_LOOP('',(#22193,#22194,#22195,#22196));
#5443=EDGE_LOOP('',(#22197,#22198,#22199,#22200));
#5444=EDGE_LOOP('',(#22201,#22202,#22203));
#5445=EDGE_LOOP('',(#22204,#22205,#22206,#22207));
#5446=EDGE_LOOP('',(#22208,#22209,#22210,#22211));
#5447=EDGE_LOOP('',(#22212,#22213,#22214));
#5448=EDGE_LOOP('',(#22215,#22216,#22217,#22218));
#5449=EDGE_LOOP('',(#22219,#22220,#22221,#22222));
#5450=EDGE_LOOP('',(#22223,#22224,#22225));
#5451=EDGE_LOOP('',(#22226,#22227,#22228,#22229));
#5452=EDGE_LOOP('',(#22230,#22231,#22232,#22233));
#5453=EDGE_LOOP('',(#22234,#22235,#22236));
#5454=EDGE_LOOP('',(#22237,#22238,#22239,#22240));
#5455=EDGE_LOOP('',(#22241,#22242,#22243,#22244));
#5456=EDGE_LOOP('',(#22245,#22246,#22247));
#5457=EDGE_LOOP('',(#22248,#22249,#22250,#22251));
#5458=EDGE_LOOP('',(#22252,#22253,#22254,#22255));
#5459=EDGE_LOOP('',(#22256,#22257,#22258));
#5460=EDGE_LOOP('',(#22259,#22260,#22261,#22262));
#5461=EDGE_LOOP('',(#22263,#22264,#22265,#22266));
#5462=EDGE_LOOP('',(#22267,#22268,#22269));
#5463=EDGE_LOOP('',(#22270,#22271,#22272,#22273));
#5464=EDGE_LOOP('',(#22274,#22275,#22276,#22277));
#5465=EDGE_LOOP('',(#22278,#22279,#22280));
#5466=EDGE_LOOP('',(#22281,#22282,#22283,#22284));
#5467=EDGE_LOOP('',(#22285,#22286,#22287,#22288));
#5468=EDGE_LOOP('',(#22289,#22290,#22291));
#5469=EDGE_LOOP('',(#22292,#22293,#22294,#22295));
#5470=EDGE_LOOP('',(#22296,#22297,#22298,#22299));
#5471=EDGE_LOOP('',(#22300,#22301,#22302,#22303));
#5472=EDGE_LOOP('',(#22304,#22305,#22306,#22307));
#5473=EDGE_LOOP('',(#22308,#22309,#22310,#22311));
#5474=EDGE_LOOP('',(#22312,#22313,#22314));
#5475=EDGE_LOOP('',(#22315,#22316,#22317,#22318));
#5476=EDGE_LOOP('',(#22319,#22320,#22321,#22322));
#5477=EDGE_LOOP('',(#22323,#22324,#22325));
#5478=EDGE_LOOP('',(#22326,#22327,#22328,#22329));
#5479=EDGE_LOOP('',(#22330,#22331,#22332,#22333));
#5480=EDGE_LOOP('',(#22334,#22335,#22336));
#5481=EDGE_LOOP('',(#22337,#22338,#22339,#22340));
#5482=EDGE_LOOP('',(#22341,#22342,#22343,#22344));
#5483=EDGE_LOOP('',(#22345,#22346,#22347));
#5484=EDGE_LOOP('',(#22348,#22349,#22350,#22351));
#5485=EDGE_LOOP('',(#22352,#22353,#22354,#22355,#22356,#22357,#22358,#22359,
#22360,#22361,#22362,#22363,#22364,#22365,#22366,#22367,#22368,#22369,#22370,
#22371,#22372,#22373,#22374,#22375,#22376,#22377,#22378,#22379,#22380,#22381,
#22382,#22383,#22384,#22385,#22386,#22387,#22388,#22389,#22390,#22391,#22392,
#22393,#22394,#22395,#22396,#22397,#22398,#22399,#22400,#22401,#22402,#22403,
#22404,#22405,#22406,#22407,#22408,#22409,#22410,#22411,#22412,#22413,#22414,
#22415,#22416,#22417,#22418,#22419,#22420,#22421,#22422,#22423,#22424,#22425,
#22426,#22427));
#5486=EDGE_LOOP('',(#22428,#22429,#22430,#22431,#22432,#22433,#22434,#22435,
#22436,#22437,#22438,#22439,#22440,#22441,#22442,#22443,#22444,#22445,#22446,
#22447,#22448,#22449,#22450,#22451,#22452,#22453,#22454,#22455,#22456,#22457,
#22458,#22459,#22460,#22461));
#5487=EDGE_LOOP('',(#22462,#22463,#22464,#22465,#22466));
#5488=EDGE_LOOP('',(#22467,#22468,#22469,#22470));
#5489=EDGE_LOOP('',(#22471,#22472,#22473,#22474,#22475,#22476,#22477,#22478,
#22479,#22480,#22481,#22482,#22483,#22484,#22485,#22486,#22487,#22488,#22489,
#22490,#22491,#22492,#22493,#22494,#22495,#22496,#22497,#22498,#22499,#22500,
#22501,#22502,#22503,#22504));
#5490=EDGE_LOOP('',(#22505));
#5491=EDGE_LOOP('',(#22506,#22507,#22508,#22509,#22510,#22511));
#5492=EDGE_LOOP('',(#22512,#22513,#22514,#22515));
#5493=EDGE_LOOP('',(#22516));
#5494=EDGE_LOOP('',(#22517,#22518,#22519,#22520));
#5495=EDGE_LOOP('',(#22521,#22522,#22523,#22524));
#5496=EDGE_LOOP('',(#22525,#22526,#22527,#22528,#22529,#22530,#22531,#22532,
#22533,#22534,#22535,#22536,#22537,#22538,#22539,#22540,#22541,#22542,#22543,
#22544,#22545,#22546,#22547,#22548,#22549,#22550,#22551,#22552,#22553,#22554,
#22555,#22556,#22557,#22558,#22559,#22560,#22561,#22562,#22563,#22564,#22565,
#22566,#22567,#22568,#22569,#22570,#22571,#22572,#22573,#22574,#22575,#22576,
#22577,#22578,#22579,#22580,#22581));
#5497=EDGE_LOOP('',(#22582));
#7697=LINE('',#46070,#10185);
#7698=LINE('',#46097,#10186);
#7699=LINE('',#46145,#10187);
#7700=LINE('',#46193,#10188);
#7701=LINE('',#46247,#10189);
#7702=LINE('',#46295,#10190);
#7703=LINE('',#46343,#10191);
#7704=LINE('',#46397,#10192);
#7705=LINE('',#46445,#10193);
#7706=LINE('',#46493,#10194);
#7707=LINE('',#46547,#10195);
#7708=LINE('',#46595,#10196);
#7709=LINE('',#46643,#10197);
#7710=LINE('',#46691,#10198);
#7711=LINE('',#46739,#10199);
#7712=LINE('',#46787,#10200);
#7713=LINE('',#46803,#10201);
#7714=LINE('',#46828,#10202);
#7715=LINE('',#46852,#10203);
#7716=LINE('',#46878,#10204);
#7717=LINE('',#46902,#10205);
#7718=LINE('',#46926,#10206);
#7719=LINE('',#46951,#10207);
#7720=LINE('',#46976,#10208);
#7721=LINE('',#47000,#10209);
#7722=LINE('',#47025,#10210);
#7723=LINE('',#47050,#10211);
#7724=LINE('',#47074,#10212);
#7725=LINE('',#47099,#10213);
#7726=LINE('',#47124,#10214);
#7727=LINE('',#47152,#10215);
#7728=LINE('',#47154,#10216);
#7729=LINE('',#47155,#10217);
#7730=LINE('',#47159,#10218);
#7731=LINE('',#47165,#10219);
#7732=LINE('',#47173,#10220);
#7733=LINE('',#47175,#10221);
#7734=LINE('',#47176,#10222);
#7735=LINE('',#47180,#10223);
#7736=LINE('',#47186,#10224);
#7737=LINE('',#47194,#10225);
#7738=LINE('',#47196,#10226);
#7739=LINE('',#47197,#10227);
#7740=LINE('',#47201,#10228);
#7741=LINE('',#47207,#10229);
#7742=LINE('',#47215,#10230);
#7743=LINE('',#47217,#10231);
#7744=LINE('',#47218,#10232);
#7745=LINE('',#47222,#10233);
#7746=LINE('',#47228,#10234);
#7747=LINE('',#47236,#10235);
#7748=LINE('',#47238,#10236);
#7749=LINE('',#47239,#10237);
#7750=LINE('',#47243,#10238);
#7751=LINE('',#47249,#10239);
#7752=LINE('',#47257,#10240);
#7753=LINE('',#47259,#10241);
#7754=LINE('',#47260,#10242);
#7755=LINE('',#47264,#10243);
#7756=LINE('',#47270,#10244);
#7757=LINE('',#47278,#10245);
#7758=LINE('',#47280,#10246);
#7759=LINE('',#47281,#10247);
#7760=LINE('',#47285,#10248);
#7761=LINE('',#47291,#10249);
#7762=LINE('',#47299,#10250);
#7763=LINE('',#47301,#10251);
#7764=LINE('',#47302,#10252);
#7765=LINE('',#47306,#10253);
#7766=LINE('',#47312,#10254);
#7767=LINE('',#47320,#10255);
#7768=LINE('',#47322,#10256);
#7769=LINE('',#47323,#10257);
#7770=LINE('',#47327,#10258);
#7771=LINE('',#47333,#10259);
#7772=LINE('',#47341,#10260);
#7773=LINE('',#47343,#10261);
#7774=LINE('',#47344,#10262);
#7775=LINE('',#47348,#10263);
#7776=LINE('',#47354,#10264);
#7777=LINE('',#47362,#10265);
#7778=LINE('',#47364,#10266);
#7779=LINE('',#47365,#10267);
#7780=LINE('',#47369,#10268);
#7781=LINE('',#47375,#10269);
#7782=LINE('',#47383,#10270);
#7783=LINE('',#47385,#10271);
#7784=LINE('',#47386,#10272);
#7785=LINE('',#47390,#10273);
#7786=LINE('',#47396,#10274);
#7787=LINE('',#47404,#10275);
#7788=LINE('',#47406,#10276);
#7789=LINE('',#47407,#10277);
#7790=LINE('',#47411,#10278);
#7791=LINE('',#47417,#10279);
#7792=LINE('',#47425,#10280);
#7793=LINE('',#47427,#10281);
#7794=LINE('',#47428,#10282);
#7795=LINE('',#47433,#10283);
#7796=LINE('',#47440,#10284);
#7797=LINE('',#47448,#10285);
#7798=LINE('',#47450,#10286);
#7799=LINE('',#47451,#10287);
#7800=LINE('',#47455,#10288);
#7801=LINE('',#47461,#10289);
#7802=LINE('',#47469,#10290);
#7803=LINE('',#47471,#10291);
#7804=LINE('',#47472,#10292);
#7805=LINE('',#47476,#10293);
#7806=LINE('',#47482,#10294);
#7807=LINE('',#47490,#10295);
#7808=LINE('',#47492,#10296);
#7809=LINE('',#47493,#10297);
#7810=LINE('',#47497,#10298);
#7811=LINE('',#47503,#10299);
#7812=LINE('',#47511,#10300);
#7813=LINE('',#47513,#10301);
#7814=LINE('',#47514,#10302);
#7815=LINE('',#47518,#10303);
#7816=LINE('',#47524,#10304);
#7817=LINE('',#47534,#10305);
#7818=LINE('',#48675,#10306);
#7819=LINE('',#48682,#10307);
#7820=LINE('',#48686,#10308);
#10185=VECTOR('',#34350,0.4);
#10186=VECTOR('',#34355,0.4);
#10187=VECTOR('',#34358,0.4);
#10188=VECTOR('',#34361,0.4);
#10189=VECTOR('',#34364,0.4);
#10190=VECTOR('',#34367,0.4);
#10191=VECTOR('',#34370,0.4);
#10192=VECTOR('',#34373,0.4);
#10193=VECTOR('',#34376,0.4);
#10194=VECTOR('',#34379,0.4);
#10195=VECTOR('',#34382,0.4);
#10196=VECTOR('',#34385,0.4);
#10197=VECTOR('',#34388,0.4);
#10198=VECTOR('',#34391,0.4);
#10199=VECTOR('',#34394,0.4);
#10200=VECTOR('',#34397,0.322275);
#10201=VECTOR('',#34402,0.322275);
#10202=VECTOR('',#34405,0.322275);
#10203=VECTOR('',#34408,0.322275);
#10204=VECTOR('',#34411,0.322275);
#10205=VECTOR('',#34414,0.322275);
#10206=VECTOR('',#34417,0.322275);
#10207=VECTOR('',#34420,0.322275);
#10208=VECTOR('',#34423,0.322275);
#10209=VECTOR('',#34426,0.322275);
#10210=VECTOR('',#34429,0.322275);
#10211=VECTOR('',#34432,0.322275);
#10212=VECTOR('',#34435,0.322275);
#10213=VECTOR('',#34438,0.322275);
#10214=VECTOR('',#34441,0.322275);
#10215=VECTOR('',#34444,1.);
#10216=VECTOR('',#34445,1.);
#10217=VECTOR('',#34446,1.);
#10218=VECTOR('',#34451,1.);
#10219=VECTOR('',#34454,1.);
#10220=VECTOR('',#34457,1.);
#10221=VECTOR('',#34458,1.);
#10222=VECTOR('',#34459,1.);
#10223=VECTOR('',#34464,1.);
#10224=VECTOR('',#34467,1.);
#10225=VECTOR('',#34470,1.);
#10226=VECTOR('',#34471,1.);
#10227=VECTOR('',#34472,1.);
#10228=VECTOR('',#34477,1.);
#10229=VECTOR('',#34480,1.);
#10230=VECTOR('',#34483,1.);
#10231=VECTOR('',#34484,1.);
#10232=VECTOR('',#34485,1.);
#10233=VECTOR('',#34490,1.);
#10234=VECTOR('',#34493,1.);
#10235=VECTOR('',#34496,1.);
#10236=VECTOR('',#34497,1.);
#10237=VECTOR('',#34498,1.);
#10238=VECTOR('',#34503,1.);
#10239=VECTOR('',#34506,1.);
#10240=VECTOR('',#34509,1.);
#10241=VECTOR('',#34510,1.);
#10242=VECTOR('',#34511,1.);
#10243=VECTOR('',#34516,1.);
#10244=VECTOR('',#34519,1.);
#10245=VECTOR('',#34522,1.);
#10246=VECTOR('',#34523,1.);
#10247=VECTOR('',#34524,1.);
#10248=VECTOR('',#34529,1.);
#10249=VECTOR('',#34532,1.);
#10250=VECTOR('',#34535,1.);
#10251=VECTOR('',#34536,1.);
#10252=VECTOR('',#34537,1.);
#10253=VECTOR('',#34542,1.);
#10254=VECTOR('',#34545,1.);
#10255=VECTOR('',#34548,1.);
#10256=VECTOR('',#34549,1.);
#10257=VECTOR('',#34550,1.);
#10258=VECTOR('',#34555,1.);
#10259=VECTOR('',#34558,1.);
#10260=VECTOR('',#34561,1.);
#10261=VECTOR('',#34562,1.);
#10262=VECTOR('',#34563,1.);
#10263=VECTOR('',#34568,1.);
#10264=VECTOR('',#34571,1.);
#10265=VECTOR('',#34574,1.);
#10266=VECTOR('',#34575,1.);
#10267=VECTOR('',#34576,1.);
#10268=VECTOR('',#34581,1.);
#10269=VECTOR('',#34584,1.);
#10270=VECTOR('',#34587,1.);
#10271=VECTOR('',#34588,1.);
#10272=VECTOR('',#34589,1.);
#10273=VECTOR('',#34594,1.);
#10274=VECTOR('',#34597,1.);
#10275=VECTOR('',#34600,1.);
#10276=VECTOR('',#34601,1.);
#10277=VECTOR('',#34602,1.);
#10278=VECTOR('',#34607,1.);
#10279=VECTOR('',#34610,1.);
#10280=VECTOR('',#34613,1.);
#10281=VECTOR('',#34614,1.);
#10282=VECTOR('',#34615,1.);
#10283=VECTOR('',#34620,1.);
#10284=VECTOR('',#34625,1.);
#10285=VECTOR('',#34628,1.);
#10286=VECTOR('',#34629,1.);
#10287=VECTOR('',#34630,1.);
#10288=VECTOR('',#34635,1.);
#10289=VECTOR('',#34638,1.);
#10290=VECTOR('',#34641,1.);
#10291=VECTOR('',#34642,1.);
#10292=VECTOR('',#34643,1.);
#10293=VECTOR('',#34648,1.);
#10294=VECTOR('',#34651,1.);
#10295=VECTOR('',#34654,1.);
#10296=VECTOR('',#34655,1.);
#10297=VECTOR('',#34656,1.);
#10298=VECTOR('',#34661,1.);
#10299=VECTOR('',#34664,1.);
#10300=VECTOR('',#34667,1.);
#10301=VECTOR('',#34668,1.);
#10302=VECTOR('',#34669,1.);
#10303=VECTOR('',#34674,1.);
#10304=VECTOR('',#34677,1.);
#10305=VECTOR('',#34694,1.1);
#10306=VECTOR('',#34735,0.375);
#10307=VECTOR('',#34746,1.);
#10308=VECTOR('',#34751,1.05);
#12551=VERTEX_POINT('',#46068);
#12552=VERTEX_POINT('',#46069);
#12553=VERTEX_POINT('',#46071);
#12554=VERTEX_POINT('',#46082);
#12555=VERTEX_POINT('',#46095);
#12556=VERTEX_POINT('',#46096);
#12557=VERTEX_POINT('',#46143);
#12558=VERTEX_POINT('',#46144);
#12559=VERTEX_POINT('',#46191);
#12560=VERTEX_POINT('',#46192);
#12561=VERTEX_POINT('',#46245);
#12562=VERTEX_POINT('',#46246);
#12563=VERTEX_POINT('',#46293);
#12564=VERTEX_POINT('',#46294);
#12565=VERTEX_POINT('',#46341);
#12566=VERTEX_POINT('',#46342);
#12567=VERTEX_POINT('',#46395);
#12568=VERTEX_POINT('',#46396);
#12569=VERTEX_POINT('',#46443);
#12570=VERTEX_POINT('',#46444);
#12571=VERTEX_POINT('',#46491);
#12572=VERTEX_POINT('',#46492);
#12573=VERTEX_POINT('',#46545);
#12574=VERTEX_POINT('',#46546);
#12575=VERTEX_POINT('',#46593);
#12576=VERTEX_POINT('',#46594);
#12577=VERTEX_POINT('',#46641);
#12578=VERTEX_POINT('',#46642);
#12579=VERTEX_POINT('',#46689);
#12580=VERTEX_POINT('',#46690);
#12581=VERTEX_POINT('',#46737);
#12582=VERTEX_POINT('',#46738);
#12583=VERTEX_POINT('',#46785);
#12584=VERTEX_POINT('',#46786);
#12585=VERTEX_POINT('',#46788);
#12586=VERTEX_POINT('',#46794);
#12587=VERTEX_POINT('',#46801);
#12588=VERTEX_POINT('',#46802);
#12589=VERTEX_POINT('',#46826);
#12590=VERTEX_POINT('',#46827);
#12591=VERTEX_POINT('',#46850);
#12592=VERTEX_POINT('',#46851);
#12593=VERTEX_POINT('',#46876);
#12594=VERTEX_POINT('',#46877);
#12595=VERTEX_POINT('',#46900);
#12596=VERTEX_POINT('',#46901);
#12597=VERTEX_POINT('',#46924);
#12598=VERTEX_POINT('',#46925);
#12599=VERTEX_POINT('',#46949);
#12600=VERTEX_POINT('',#46950);
#12601=VERTEX_POINT('',#46974);
#12602=VERTEX_POINT('',#46975);
#12603=VERTEX_POINT('',#46998);
#12604=VERTEX_POINT('',#46999);
#12605=VERTEX_POINT('',#47023);
#12606=VERTEX_POINT('',#47024);
#12607=VERTEX_POINT('',#47048);
#12608=VERTEX_POINT('',#47049);
#12609=VERTEX_POINT('',#47072);
#12610=VERTEX_POINT('',#47073);
#12611=VERTEX_POINT('',#47097);
#12612=VERTEX_POINT('',#47098);
#12613=VERTEX_POINT('',#47122);
#12614=VERTEX_POINT('',#47123);
#12615=VERTEX_POINT('',#47146);
#12616=VERTEX_POINT('',#47147);
#12617=VERTEX_POINT('',#47151);
#12618=VERTEX_POINT('',#47153);
#12619=VERTEX_POINT('',#47157);
#12620=VERTEX_POINT('',#47161);
#12621=VERTEX_POINT('',#47167);
#12622=VERTEX_POINT('',#47168);
#12623=VERTEX_POINT('',#47172);
#12624=VERTEX_POINT('',#47174);
#12625=VERTEX_POINT('',#47178);
#12626=VERTEX_POINT('',#47182);
#12627=VERTEX_POINT('',#47188);
#12628=VERTEX_POINT('',#47189);
#12629=VERTEX_POINT('',#47193);
#12630=VERTEX_POINT('',#47195);
#12631=VERTEX_POINT('',#47199);
#12632=VERTEX_POINT('',#47203);
#12633=VERTEX_POINT('',#47209);
#12634=VERTEX_POINT('',#47210);
#12635=VERTEX_POINT('',#47214);
#12636=VERTEX_POINT('',#47216);
#12637=VERTEX_POINT('',#47220);
#12638=VERTEX_POINT('',#47224);
#12639=VERTEX_POINT('',#47230);
#12640=VERTEX_POINT('',#47231);
#12641=VERTEX_POINT('',#47235);
#12642=VERTEX_POINT('',#47237);
#12643=VERTEX_POINT('',#47241);
#12644=VERTEX_POINT('',#47245);
#12645=VERTEX_POINT('',#47251);
#12646=VERTEX_POINT('',#47252);
#12647=VERTEX_POINT('',#47256);
#12648=VERTEX_POINT('',#47258);
#12649=VERTEX_POINT('',#47262);
#12650=VERTEX_POINT('',#47266);
#12651=VERTEX_POINT('',#47272);
#12652=VERTEX_POINT('',#47273);
#12653=VERTEX_POINT('',#47277);
#12654=VERTEX_POINT('',#47279);
#12655=VERTEX_POINT('',#47283);
#12656=VERTEX_POINT('',#47287);
#12657=VERTEX_POINT('',#47293);
#12658=VERTEX_POINT('',#47294);
#12659=VERTEX_POINT('',#47298);
#12660=VERTEX_POINT('',#47300);
#12661=VERTEX_POINT('',#47304);
#12662=VERTEX_POINT('',#47308);
#12663=VERTEX_POINT('',#47314);
#12664=VERTEX_POINT('',#47315);
#12665=VERTEX_POINT('',#47319);
#12666=VERTEX_POINT('',#47321);
#12667=VERTEX_POINT('',#47325);
#12668=VERTEX_POINT('',#47329);
#12669=VERTEX_POINT('',#47335);
#12670=VERTEX_POINT('',#47336);
#12671=VERTEX_POINT('',#47340);
#12672=VERTEX_POINT('',#47342);
#12673=VERTEX_POINT('',#47346);
#12674=VERTEX_POINT('',#47350);
#12675=VERTEX_POINT('',#47356);
#12676=VERTEX_POINT('',#47357);
#12677=VERTEX_POINT('',#47361);
#12678=VERTEX_POINT('',#47363);
#12679=VERTEX_POINT('',#47367);
#12680=VERTEX_POINT('',#47371);
#12681=VERTEX_POINT('',#47377);
#12682=VERTEX_POINT('',#47378);
#12683=VERTEX_POINT('',#47382);
#12684=VERTEX_POINT('',#47384);
#12685=VERTEX_POINT('',#47388);
#12686=VERTEX_POINT('',#47392);
#12687=VERTEX_POINT('',#47398);
#12688=VERTEX_POINT('',#47399);
#12689=VERTEX_POINT('',#47403);
#12690=VERTEX_POINT('',#47405);
#12691=VERTEX_POINT('',#47409);
#12692=VERTEX_POINT('',#47413);
#12693=VERTEX_POINT('',#47419);
#12694=VERTEX_POINT('',#47420);
#12695=VERTEX_POINT('',#47424);
#12696=VERTEX_POINT('',#47426);
#12697=VERTEX_POINT('',#47430);
#12698=VERTEX_POINT('',#47432);
#12699=VERTEX_POINT('',#47436);
#12700=VERTEX_POINT('',#47442);
#12701=VERTEX_POINT('',#47443);
#12702=VERTEX_POINT('',#47447);
#12703=VERTEX_POINT('',#47449);
#12704=VERTEX_POINT('',#47453);
#12705=VERTEX_POINT('',#47457);
#12706=VERTEX_POINT('',#47463);
#12707=VERTEX_POINT('',#47464);
#12708=VERTEX_POINT('',#47468);
#12709=VERTEX_POINT('',#47470);
#12710=VERTEX_POINT('',#47474);
#12711=VERTEX_POINT('',#47478);
#12712=VERTEX_POINT('',#47484);
#12713=VERTEX_POINT('',#47485);
#12714=VERTEX_POINT('',#47489);
#12715=VERTEX_POINT('',#47491);
#12716=VERTEX_POINT('',#47495);
#12717=VERTEX_POINT('',#47499);
#12718=VERTEX_POINT('',#47505);
#12719=VERTEX_POINT('',#47506);
#12720=VERTEX_POINT('',#47510);
#12721=VERTEX_POINT('',#47512);
#12722=VERTEX_POINT('',#47516);
#12723=VERTEX_POINT('',#47520);
#12724=VERTEX_POINT('',#47533);
#12725=VERTEX_POINT('',#47951);
#12726=VERTEX_POINT('',#48032);
#12727=VERTEX_POINT('',#48107);
#12728=VERTEX_POINT('',#48110);
#12729=VERTEX_POINT('',#48590);
#12730=VERTEX_POINT('',#48672);
#12731=VERTEX_POINT('',#48679);
#12732=VERTEX_POINT('',#48684);
#15900=EDGE_CURVE('',#12551,#12552,#7697,.T.);
#15901=EDGE_CURVE('',#12551,#12553,#810,.T.);
#15902=EDGE_CURVE('',#12553,#12554,#2400,.T.);
#15903=EDGE_CURVE('',#12554,#12552,#811,.T.);
#15904=EDGE_CURVE('',#12555,#12556,#7698,.T.);
#15905=EDGE_CURVE('',#12555,#12551,#812,.T.);
#15906=EDGE_CURVE('',#12552,#12556,#813,.T.);
#15907=EDGE_CURVE('',#12557,#12558,#7699,.T.);
#15908=EDGE_CURVE('',#12557,#12555,#814,.T.);
#15909=EDGE_CURVE('',#12556,#12558,#815,.T.);
#15910=EDGE_CURVE('',#12559,#12560,#7700,.T.);
#15911=EDGE_CURVE('',#12559,#12557,#816,.T.);
#15912=EDGE_CURVE('',#12558,#12560,#817,.T.);
#15913=EDGE_CURVE('',#12561,#12562,#7701,.T.);
#15914=EDGE_CURVE('',#12561,#12559,#818,.T.);
#15915=EDGE_CURVE('',#12560,#12562,#819,.T.);
#15916=EDGE_CURVE('',#12563,#12564,#7702,.T.);
#15917=EDGE_CURVE('',#12563,#12561,#820,.T.);
#15918=EDGE_CURVE('',#12562,#12564,#821,.T.);
#15919=EDGE_CURVE('',#12565,#12566,#7703,.T.);
#15920=EDGE_CURVE('',#12565,#12563,#822,.T.);
#15921=EDGE_CURVE('',#12564,#12566,#823,.T.);
#15922=EDGE_CURVE('',#12567,#12568,#7704,.T.);
#15923=EDGE_CURVE('',#12567,#12565,#824,.T.);
#15924=EDGE_CURVE('',#12566,#12568,#825,.T.);
#15925=EDGE_CURVE('',#12569,#12570,#7705,.T.);
#15926=EDGE_CURVE('',#12569,#12567,#826,.T.);
#15927=EDGE_CURVE('',#12568,#12570,#827,.T.);
#15928=EDGE_CURVE('',#12571,#12572,#7706,.T.);
#15929=EDGE_CURVE('',#12571,#12569,#828,.T.);
#15930=EDGE_CURVE('',#12570,#12572,#829,.T.);
#15931=EDGE_CURVE('',#12573,#12574,#7707,.T.);
#15932=EDGE_CURVE('',#12573,#12571,#830,.T.);
#15933=EDGE_CURVE('',#12572,#12574,#831,.T.);
#15934=EDGE_CURVE('',#12575,#12576,#7708,.T.);
#15935=EDGE_CURVE('',#12575,#12573,#832,.T.);
#15936=EDGE_CURVE('',#12574,#12576,#833,.T.);
#15937=EDGE_CURVE('',#12577,#12578,#7709,.T.);
#15938=EDGE_CURVE('',#12577,#12575,#834,.T.);
#15939=EDGE_CURVE('',#12576,#12578,#835,.T.);
#15940=EDGE_CURVE('',#12579,#12580,#7710,.T.);
#15941=EDGE_CURVE('',#12579,#12577,#836,.T.);
#15942=EDGE_CURVE('',#12578,#12580,#837,.T.);
#15943=EDGE_CURVE('',#12581,#12582,#7711,.T.);
#15944=EDGE_CURVE('',#12581,#12579,#838,.T.);
#15945=EDGE_CURVE('',#12580,#12582,#839,.T.);
#15946=EDGE_CURVE('',#12583,#12584,#7712,.T.);
#15947=EDGE_CURVE('',#12583,#12585,#840,.T.);
#15948=EDGE_CURVE('',#12586,#12585,#2401,.T.);
#15949=EDGE_CURVE('',#12584,#12586,#841,.T.);
#15950=EDGE_CURVE('',#12587,#12588,#7713,.T.);
#15951=EDGE_CURVE('',#12587,#12583,#842,.T.);
#15952=EDGE_CURVE('',#12588,#12584,#843,.T.);
#15953=EDGE_CURVE('',#12589,#12590,#7714,.T.);
#15954=EDGE_CURVE('',#12589,#12587,#844,.T.);
#15955=EDGE_CURVE('',#12590,#12588,#845,.T.);
#15956=EDGE_CURVE('',#12591,#12592,#7715,.T.);
#15957=EDGE_CURVE('',#12591,#12589,#846,.T.);
#15958=EDGE_CURVE('',#12592,#12590,#847,.T.);
#15959=EDGE_CURVE('',#12593,#12594,#7716,.T.);
#15960=EDGE_CURVE('',#12593,#12591,#848,.T.);
#15961=EDGE_CURVE('',#12594,#12592,#849,.T.);
#15962=EDGE_CURVE('',#12595,#12596,#7717,.T.);
#15963=EDGE_CURVE('',#12595,#12593,#850,.T.);
#15964=EDGE_CURVE('',#12596,#12594,#851,.T.);
#15965=EDGE_CURVE('',#12597,#12598,#7718,.T.);
#15966=EDGE_CURVE('',#12597,#12595,#852,.T.);
#15967=EDGE_CURVE('',#12598,#12596,#853,.T.);
#15968=EDGE_CURVE('',#12599,#12600,#7719,.T.);
#15969=EDGE_CURVE('',#12599,#12597,#854,.T.);
#15970=EDGE_CURVE('',#12600,#12598,#855,.T.);
#15971=EDGE_CURVE('',#12601,#12602,#7720,.T.);
#15972=EDGE_CURVE('',#12601,#12599,#856,.T.);
#15973=EDGE_CURVE('',#12602,#12600,#857,.T.);
#15974=EDGE_CURVE('',#12603,#12604,#7721,.T.);
#15975=EDGE_CURVE('',#12603,#12601,#858,.T.);
#15976=EDGE_CURVE('',#12604,#12602,#859,.T.);
#15977=EDGE_CURVE('',#12605,#12606,#7722,.T.);
#15978=EDGE_CURVE('',#12605,#12603,#860,.T.);
#15979=EDGE_CURVE('',#12606,#12604,#861,.T.);
#15980=EDGE_CURVE('',#12607,#12608,#7723,.T.);
#15981=EDGE_CURVE('',#12607,#12605,#862,.T.);
#15982=EDGE_CURVE('',#12608,#12606,#863,.T.);
#15983=EDGE_CURVE('',#12609,#12610,#7724,.T.);
#15984=EDGE_CURVE('',#12609,#12607,#864,.T.);
#15985=EDGE_CURVE('',#12610,#12608,#865,.T.);
#15986=EDGE_CURVE('',#12611,#12612,#7725,.T.);
#15987=EDGE_CURVE('',#12611,#12609,#866,.T.);
#15988=EDGE_CURVE('',#12612,#12610,#867,.T.);
#15989=EDGE_CURVE('',#12613,#12614,#7726,.T.);
#15990=EDGE_CURVE('',#12613,#12611,#868,.T.);
#15991=EDGE_CURVE('',#12614,#12612,#869,.T.);
#15992=EDGE_CURVE('',#12615,#12616,#319,.T.);
#15993=EDGE_CURVE('',#12615,#12617,#7727,.T.);
#15994=EDGE_CURVE('',#12617,#12618,#7728,.T.);
#15995=EDGE_CURVE('',#12616,#12618,#7729,.T.);
#15996=EDGE_CURVE('',#12618,#12619,#2402,.T.);
#15997=EDGE_CURVE('',#12619,#12617,#7730,.T.);
#15998=EDGE_CURVE('',#12620,#12615,#320,.T.);
#15999=EDGE_CURVE('',#12619,#12620,#7731,.T.);
#16000=EDGE_CURVE('',#12621,#12622,#321,.T.);
#16001=EDGE_CURVE('',#12621,#12623,#7732,.T.);
#16002=EDGE_CURVE('',#12623,#12624,#7733,.T.);
#16003=EDGE_CURVE('',#12622,#12624,#7734,.T.);
#16004=EDGE_CURVE('',#12624,#12625,#2403,.T.);
#16005=EDGE_CURVE('',#12625,#12623,#7735,.T.);
#16006=EDGE_CURVE('',#12626,#12621,#322,.T.);
#16007=EDGE_CURVE('',#12625,#12626,#7736,.T.);
#16008=EDGE_CURVE('',#12627,#12628,#323,.T.);
#16009=EDGE_CURVE('',#12627,#12629,#7737,.T.);
#16010=EDGE_CURVE('',#12629,#12630,#7738,.T.);
#16011=EDGE_CURVE('',#12628,#12630,#7739,.T.);
#16012=EDGE_CURVE('',#12630,#12631,#2404,.T.);
#16013=EDGE_CURVE('',#12631,#12629,#7740,.T.);
#16014=EDGE_CURVE('',#12632,#12627,#324,.T.);
#16015=EDGE_CURVE('',#12631,#12632,#7741,.T.);
#16016=EDGE_CURVE('',#12633,#12634,#325,.T.);
#16017=EDGE_CURVE('',#12633,#12635,#7742,.T.);
#16018=EDGE_CURVE('',#12635,#12636,#7743,.T.);
#16019=EDGE_CURVE('',#12634,#12636,#7744,.T.);
#16020=EDGE_CURVE('',#12636,#12637,#2405,.T.);
#16021=EDGE_CURVE('',#12637,#12635,#7745,.T.);
#16022=EDGE_CURVE('',#12638,#12633,#326,.T.);
#16023=EDGE_CURVE('',#12637,#12638,#7746,.T.);
#16024=EDGE_CURVE('',#12639,#12640,#327,.T.);
#16025=EDGE_CURVE('',#12639,#12641,#7747,.T.);
#16026=EDGE_CURVE('',#12641,#12642,#7748,.T.);
#16027=EDGE_CURVE('',#12640,#12642,#7749,.T.);
#16028=EDGE_CURVE('',#12642,#12643,#2406,.T.);
#16029=EDGE_CURVE('',#12643,#12641,#7750,.T.);
#16030=EDGE_CURVE('',#12644,#12639,#328,.T.);
#16031=EDGE_CURVE('',#12643,#12644,#7751,.T.);
#16032=EDGE_CURVE('',#12645,#12646,#329,.T.);
#16033=EDGE_CURVE('',#12645,#12647,#7752,.T.);
#16034=EDGE_CURVE('',#12647,#12648,#7753,.T.);
#16035=EDGE_CURVE('',#12646,#12648,#7754,.T.);
#16036=EDGE_CURVE('',#12648,#12649,#2407,.T.);
#16037=EDGE_CURVE('',#12649,#12647,#7755,.T.);
#16038=EDGE_CURVE('',#12650,#12645,#330,.T.);
#16039=EDGE_CURVE('',#12649,#12650,#7756,.T.);
#16040=EDGE_CURVE('',#12651,#12652,#331,.T.);
#16041=EDGE_CURVE('',#12651,#12653,#7757,.T.);
#16042=EDGE_CURVE('',#12653,#12654,#7758,.T.);
#16043=EDGE_CURVE('',#12652,#12654,#7759,.T.);
#16044=EDGE_CURVE('',#12654,#12655,#2408,.T.);
#16045=EDGE_CURVE('',#12655,#12653,#7760,.T.);
#16046=EDGE_CURVE('',#12656,#12651,#332,.T.);
#16047=EDGE_CURVE('',#12655,#12656,#7761,.T.);
#16048=EDGE_CURVE('',#12657,#12658,#333,.T.);
#16049=EDGE_CURVE('',#12657,#12659,#7762,.T.);
#16050=EDGE_CURVE('',#12659,#12660,#7763,.T.);
#16051=EDGE_CURVE('',#12658,#12660,#7764,.T.);
#16052=EDGE_CURVE('',#12660,#12661,#2409,.T.);
#16053=EDGE_CURVE('',#12661,#12659,#7765,.T.);
#16054=EDGE_CURVE('',#12662,#12657,#334,.T.);
#16055=EDGE_CURVE('',#12661,#12662,#7766,.T.);
#16056=EDGE_CURVE('',#12663,#12664,#335,.T.);
#16057=EDGE_CURVE('',#12663,#12665,#7767,.T.);
#16058=EDGE_CURVE('',#12665,#12666,#7768,.T.);
#16059=EDGE_CURVE('',#12664,#12666,#7769,.T.);
#16060=EDGE_CURVE('',#12666,#12667,#2410,.T.);
#16061=EDGE_CURVE('',#12667,#12665,#7770,.T.);
#16062=EDGE_CURVE('',#12668,#12663,#336,.T.);
#16063=EDGE_CURVE('',#12667,#12668,#7771,.T.);
#16064=EDGE_CURVE('',#12669,#12670,#337,.T.);
#16065=EDGE_CURVE('',#12669,#12671,#7772,.T.);
#16066=EDGE_CURVE('',#12671,#12672,#7773,.T.);
#16067=EDGE_CURVE('',#12670,#12672,#7774,.T.);
#16068=EDGE_CURVE('',#12672,#12673,#2411,.T.);
#16069=EDGE_CURVE('',#12673,#12671,#7775,.T.);
#16070=EDGE_CURVE('',#12674,#12669,#338,.T.);
#16071=EDGE_CURVE('',#12673,#12674,#7776,.T.);
#16072=EDGE_CURVE('',#12675,#12676,#339,.T.);
#16073=EDGE_CURVE('',#12675,#12677,#7777,.T.);
#16074=EDGE_CURVE('',#12677,#12678,#7778,.T.);
#16075=EDGE_CURVE('',#12676,#12678,#7779,.T.);
#16076=EDGE_CURVE('',#12678,#12679,#2412,.T.);
#16077=EDGE_CURVE('',#12679,#12677,#7780,.T.);
#16078=EDGE_CURVE('',#12680,#12675,#340,.T.);
#16079=EDGE_CURVE('',#12679,#12680,#7781,.T.);
#16080=EDGE_CURVE('',#12681,#12682,#341,.T.);
#16081=EDGE_CURVE('',#12681,#12683,#7782,.T.);
#16082=EDGE_CURVE('',#12683,#12684,#7783,.T.);
#16083=EDGE_CURVE('',#12682,#12684,#7784,.T.);
#16084=EDGE_CURVE('',#12684,#12685,#2413,.T.);
#16085=EDGE_CURVE('',#12685,#12683,#7785,.T.);
#16086=EDGE_CURVE('',#12686,#12681,#342,.T.);
#16087=EDGE_CURVE('',#12685,#12686,#7786,.T.);
#16088=EDGE_CURVE('',#12687,#12688,#343,.T.);
#16089=EDGE_CURVE('',#12687,#12689,#7787,.T.);
#16090=EDGE_CURVE('',#12689,#12690,#7788,.T.);
#16091=EDGE_CURVE('',#12688,#12690,#7789,.T.);
#16092=EDGE_CURVE('',#12690,#12691,#2414,.T.);
#16093=EDGE_CURVE('',#12691,#12689,#7790,.T.);
#16094=EDGE_CURVE('',#12692,#12687,#344,.T.);
#16095=EDGE_CURVE('',#12691,#12692,#7791,.T.);
#16096=EDGE_CURVE('',#12693,#12694,#345,.T.);
#16097=EDGE_CURVE('',#12693,#12695,#7792,.T.);
#16098=EDGE_CURVE('',#12695,#12696,#7793,.T.);
#16099=EDGE_CURVE('',#12694,#12696,#7794,.T.);
#16100=EDGE_CURVE('',#12696,#12697,#2415,.T.);
#16101=EDGE_CURVE('',#12698,#12695,#7795,.T.);
#16102=EDGE_CURVE('',#12697,#12698,#2416,.T.);
#16103=EDGE_CURVE('',#12699,#12693,#346,.T.);
#16104=EDGE_CURVE('',#12698,#12699,#7796,.T.);
#16105=EDGE_CURVE('',#12700,#12701,#347,.T.);
#16106=EDGE_CURVE('',#12700,#12702,#7797,.T.);
#16107=EDGE_CURVE('',#12702,#12703,#7798,.T.);
#16108=EDGE_CURVE('',#12701,#12703,#7799,.T.);
#16109=EDGE_CURVE('',#12703,#12704,#2417,.T.);
#16110=EDGE_CURVE('',#12704,#12702,#7800,.T.);
#16111=EDGE_CURVE('',#12705,#12700,#348,.T.);
#16112=EDGE_CURVE('',#12704,#12705,#7801,.T.);
#16113=EDGE_CURVE('',#12706,#12707,#349,.T.);
#16114=EDGE_CURVE('',#12706,#12708,#7802,.T.);
#16115=EDGE_CURVE('',#12708,#12709,#7803,.T.);
#16116=EDGE_CURVE('',#12707,#12709,#7804,.T.);
#16117=EDGE_CURVE('',#12709,#12710,#2418,.T.);
#16118=EDGE_CURVE('',#12710,#12708,#7805,.T.);
#16119=EDGE_CURVE('',#12711,#12706,#350,.T.);
#16120=EDGE_CURVE('',#12710,#12711,#7806,.T.);
#16121=EDGE_CURVE('',#12712,#12713,#351,.T.);
#16122=EDGE_CURVE('',#12712,#12714,#7807,.T.);
#16123=EDGE_CURVE('',#12714,#12715,#7808,.T.);
#16124=EDGE_CURVE('',#12713,#12715,#7809,.T.);
#16125=EDGE_CURVE('',#12715,#12716,#2419,.T.);
#16126=EDGE_CURVE('',#12716,#12714,#7810,.T.);
#16127=EDGE_CURVE('',#12717,#12712,#352,.T.);
#16128=EDGE_CURVE('',#12716,#12717,#7811,.T.);
#16129=EDGE_CURVE('',#12718,#12719,#353,.T.);
#16130=EDGE_CURVE('',#12718,#12720,#7812,.T.);
#16131=EDGE_CURVE('',#12720,#12721,#7813,.T.);
#16132=EDGE_CURVE('',#12719,#12721,#7814,.T.);
#16133=EDGE_CURVE('',#12721,#12722,#2420,.T.);
#16134=EDGE_CURVE('',#12722,#12720,#7815,.T.);
#16135=EDGE_CURVE('',#12723,#12718,#354,.T.);
#16136=EDGE_CURVE('',#12722,#12723,#7816,.T.);
#16137=EDGE_CURVE('',#12713,#12620,#2421,.T.);
#16138=EDGE_CURVE('',#12622,#12717,#2422,.T.);
#16139=EDGE_CURVE('',#12707,#12626,#2423,.T.);
#16140=EDGE_CURVE('',#12628,#12711,#2424,.T.);
#16141=EDGE_CURVE('',#12701,#12632,#2425,.T.);
#16142=EDGE_CURVE('',#12634,#12705,#2426,.T.);
#16143=EDGE_CURVE('',#12694,#12638,#2427,.T.);
#16144=EDGE_CURVE('',#12697,#12724,#7817,.T.);
#16145=EDGE_CURVE('',#12724,#12724,#2428,.T.);
#16146=EDGE_CURVE('',#12688,#12699,#2429,.T.);
#16147=EDGE_CURVE('',#12646,#12692,#2430,.T.);
#16148=EDGE_CURVE('',#12682,#12650,#2431,.T.);
#16149=EDGE_CURVE('',#12652,#12686,#2432,.T.);
#16150=EDGE_CURVE('',#12676,#12656,#2433,.T.);
#16151=EDGE_CURVE('',#12658,#12680,#2434,.T.);
#16152=EDGE_CURVE('',#12670,#12662,#2435,.T.);
#16153=EDGE_CURVE('',#12664,#12674,#2436,.T.);
#16154=EDGE_CURVE('',#12640,#12668,#2437,.T.);
#16155=EDGE_CURVE('',#12719,#12644,#2438,.T.);
#16156=EDGE_CURVE('',#12616,#12723,#2439,.T.);
#16157=EDGE_CURVE('',#12725,#12586,#870,.T.);
#16158=EDGE_CURVE('',#12582,#12725,#871,.T.);
#16159=EDGE_CURVE('',#12726,#12554,#872,.T.);
#16160=EDGE_CURVE('',#12726,#12614,#873,.T.);
#16161=EDGE_CURVE('',#12554,#12727,#2440,.T.);
#16162=EDGE_CURVE('',#12727,#12553,#2441,.T.);
#16163=EDGE_CURVE('',#12553,#12728,#874,.T.);
#16164=EDGE_CURVE('',#12728,#12726,#2442,.T.);
#16165=EDGE_CURVE('',#12728,#12613,#875,.T.);
#16166=EDGE_CURVE('',#12585,#12729,#876,.T.);
#16167=EDGE_CURVE('',#12729,#12581,#877,.T.);
#16168=EDGE_CURVE('',#12730,#12730,#2443,.T.);
#16169=EDGE_CURVE('',#12727,#12730,#7818,.T.);
#16170=EDGE_CURVE('',#12729,#12725,#2444,.T.);
#16171=EDGE_CURVE('',#12731,#12731,#2445,.T.);
#16172=EDGE_CURVE('',#12724,#12731,#7819,.T.);
#16173=EDGE_CURVE('',#12732,#12732,#2446,.T.);
#16174=EDGE_CURVE('',#12732,#12693,#7820,.T.);
#22033=ORIENTED_EDGE('',*,*,#15900,.F.);
#22034=ORIENTED_EDGE('',*,*,#15901,.T.);
#22035=ORIENTED_EDGE('',*,*,#15902,.T.);
#22036=ORIENTED_EDGE('',*,*,#15903,.T.);
#22037=ORIENTED_EDGE('',*,*,#15904,.F.);
#22038=ORIENTED_EDGE('',*,*,#15905,.T.);
#22039=ORIENTED_EDGE('',*,*,#15900,.T.);
#22040=ORIENTED_EDGE('',*,*,#15906,.T.);
#22041=ORIENTED_EDGE('',*,*,#15907,.F.);
#22042=ORIENTED_EDGE('',*,*,#15908,.T.);
#22043=ORIENTED_EDGE('',*,*,#15904,.T.);
#22044=ORIENTED_EDGE('',*,*,#15909,.T.);
#22045=ORIENTED_EDGE('',*,*,#15910,.F.);
#22046=ORIENTED_EDGE('',*,*,#15911,.T.);
#22047=ORIENTED_EDGE('',*,*,#15907,.T.);
#22048=ORIENTED_EDGE('',*,*,#15912,.T.);
#22049=ORIENTED_EDGE('',*,*,#15913,.F.);
#22050=ORIENTED_EDGE('',*,*,#15914,.T.);
#22051=ORIENTED_EDGE('',*,*,#15910,.T.);
#22052=ORIENTED_EDGE('',*,*,#15915,.T.);
#22053=ORIENTED_EDGE('',*,*,#15916,.F.);
#22054=ORIENTED_EDGE('',*,*,#15917,.T.);
#22055=ORIENTED_EDGE('',*,*,#15913,.T.);
#22056=ORIENTED_EDGE('',*,*,#15918,.T.);
#22057=ORIENTED_EDGE('',*,*,#15919,.F.);
#22058=ORIENTED_EDGE('',*,*,#15920,.T.);
#22059=ORIENTED_EDGE('',*,*,#15916,.T.);
#22060=ORIENTED_EDGE('',*,*,#15921,.T.);
#22061=ORIENTED_EDGE('',*,*,#15922,.F.);
#22062=ORIENTED_EDGE('',*,*,#15923,.T.);
#22063=ORIENTED_EDGE('',*,*,#15919,.T.);
#22064=ORIENTED_EDGE('',*,*,#15924,.T.);
#22065=ORIENTED_EDGE('',*,*,#15925,.F.);
#22066=ORIENTED_EDGE('',*,*,#15926,.T.);
#22067=ORIENTED_EDGE('',*,*,#15922,.T.);
#22068=ORIENTED_EDGE('',*,*,#15927,.T.);
#22069=ORIENTED_EDGE('',*,*,#15928,.F.);
#22070=ORIENTED_EDGE('',*,*,#15929,.T.);
#22071=ORIENTED_EDGE('',*,*,#15925,.T.);
#22072=ORIENTED_EDGE('',*,*,#15930,.T.);
#22073=ORIENTED_EDGE('',*,*,#15931,.F.);
#22074=ORIENTED_EDGE('',*,*,#15932,.T.);
#22075=ORIENTED_EDGE('',*,*,#15928,.T.);
#22076=ORIENTED_EDGE('',*,*,#15933,.T.);
#22077=ORIENTED_EDGE('',*,*,#15934,.F.);
#22078=ORIENTED_EDGE('',*,*,#15935,.T.);
#22079=ORIENTED_EDGE('',*,*,#15931,.T.);
#22080=ORIENTED_EDGE('',*,*,#15936,.T.);
#22081=ORIENTED_EDGE('',*,*,#15937,.F.);
#22082=ORIENTED_EDGE('',*,*,#15938,.T.);
#22083=ORIENTED_EDGE('',*,*,#15934,.T.);
#22084=ORIENTED_EDGE('',*,*,#15939,.T.);
#22085=ORIENTED_EDGE('',*,*,#15940,.F.);
#22086=ORIENTED_EDGE('',*,*,#15941,.T.);
#22087=ORIENTED_EDGE('',*,*,#15937,.T.);
#22088=ORIENTED_EDGE('',*,*,#15942,.T.);
#22089=ORIENTED_EDGE('',*,*,#15943,.F.);
#22090=ORIENTED_EDGE('',*,*,#15944,.T.);
#22091=ORIENTED_EDGE('',*,*,#15940,.T.);
#22092=ORIENTED_EDGE('',*,*,#15945,.T.);
#22093=ORIENTED_EDGE('',*,*,#15946,.F.);
#22094=ORIENTED_EDGE('',*,*,#15947,.T.);
#22095=ORIENTED_EDGE('',*,*,#15948,.F.);
#22096=ORIENTED_EDGE('',*,*,#15949,.F.);
#22097=ORIENTED_EDGE('',*,*,#15950,.F.);
#22098=ORIENTED_EDGE('',*,*,#15951,.T.);
#22099=ORIENTED_EDGE('',*,*,#15946,.T.);
#22100=ORIENTED_EDGE('',*,*,#15952,.F.);
#22101=ORIENTED_EDGE('',*,*,#15953,.F.);
#22102=ORIENTED_EDGE('',*,*,#15954,.T.);
#22103=ORIENTED_EDGE('',*,*,#15950,.T.);
#22104=ORIENTED_EDGE('',*,*,#15955,.F.);
#22105=ORIENTED_EDGE('',*,*,#15956,.F.);
#22106=ORIENTED_EDGE('',*,*,#15957,.T.);
#22107=ORIENTED_EDGE('',*,*,#15953,.T.);
#22108=ORIENTED_EDGE('',*,*,#15958,.F.);
#22109=ORIENTED_EDGE('',*,*,#15959,.F.);
#22110=ORIENTED_EDGE('',*,*,#15960,.T.);
#22111=ORIENTED_EDGE('',*,*,#15956,.T.);
#22112=ORIENTED_EDGE('',*,*,#15961,.F.);
#22113=ORIENTED_EDGE('',*,*,#15962,.F.);
#22114=ORIENTED_EDGE('',*,*,#15963,.T.);
#22115=ORIENTED_EDGE('',*,*,#15959,.T.);
#22116=ORIENTED_EDGE('',*,*,#15964,.F.);
#22117=ORIENTED_EDGE('',*,*,#15965,.F.);
#22118=ORIENTED_EDGE('',*,*,#15966,.T.);
#22119=ORIENTED_EDGE('',*,*,#15962,.T.);
#22120=ORIENTED_EDGE('',*,*,#15967,.F.);
#22121=ORIENTED_EDGE('',*,*,#15968,.F.);
#22122=ORIENTED_EDGE('',*,*,#15969,.T.);
#22123=ORIENTED_EDGE('',*,*,#15965,.T.);
#22124=ORIENTED_EDGE('',*,*,#15970,.F.);
#22125=ORIENTED_EDGE('',*,*,#15971,.F.);
#22126=ORIENTED_EDGE('',*,*,#15972,.T.);
#22127=ORIENTED_EDGE('',*,*,#15968,.T.);
#22128=ORIENTED_EDGE('',*,*,#15973,.F.);
#22129=ORIENTED_EDGE('',*,*,#15974,.F.);
#22130=ORIENTED_EDGE('',*,*,#15975,.T.);
#22131=ORIENTED_EDGE('',*,*,#15971,.T.);
#22132=ORIENTED_EDGE('',*,*,#15976,.F.);
#22133=ORIENTED_EDGE('',*,*,#15977,.F.);
#22134=ORIENTED_EDGE('',*,*,#15978,.T.);
#22135=ORIENTED_EDGE('',*,*,#15974,.T.);
#22136=ORIENTED_EDGE('',*,*,#15979,.F.);
#22137=ORIENTED_EDGE('',*,*,#15980,.F.);
#22138=ORIENTED_EDGE('',*,*,#15981,.T.);
#22139=ORIENTED_EDGE('',*,*,#15977,.T.);
#22140=ORIENTED_EDGE('',*,*,#15982,.F.);
#22141=ORIENTED_EDGE('',*,*,#15983,.F.);
#22142=ORIENTED_EDGE('',*,*,#15984,.T.);
#22143=ORIENTED_EDGE('',*,*,#15980,.T.);
#22144=ORIENTED_EDGE('',*,*,#15985,.F.);
#22145=ORIENTED_EDGE('',*,*,#15986,.F.);
#22146=ORIENTED_EDGE('',*,*,#15987,.T.);
#22147=ORIENTED_EDGE('',*,*,#15983,.T.);
#22148=ORIENTED_EDGE('',*,*,#15988,.F.);
#22149=ORIENTED_EDGE('',*,*,#15989,.F.);
#22150=ORIENTED_EDGE('',*,*,#15990,.T.);
#22151=ORIENTED_EDGE('',*,*,#15986,.T.);
#22152=ORIENTED_EDGE('',*,*,#15991,.F.);
#22153=ORIENTED_EDGE('',*,*,#15992,.F.);
#22154=ORIENTED_EDGE('',*,*,#15993,.T.);
#22155=ORIENTED_EDGE('',*,*,#15994,.T.);
#22156=ORIENTED_EDGE('',*,*,#15995,.F.);
#22157=ORIENTED_EDGE('',*,*,#15996,.F.);
#22158=ORIENTED_EDGE('',*,*,#15994,.F.);
#22159=ORIENTED_EDGE('',*,*,#15997,.F.);
#22160=ORIENTED_EDGE('',*,*,#15998,.F.);
#22161=ORIENTED_EDGE('',*,*,#15999,.F.);
#22162=ORIENTED_EDGE('',*,*,#15997,.T.);
#22163=ORIENTED_EDGE('',*,*,#15993,.F.);
#22164=ORIENTED_EDGE('',*,*,#16000,.F.);
#22165=ORIENTED_EDGE('',*,*,#16001,.T.);
#22166=ORIENTED_EDGE('',*,*,#16002,.T.);
#22167=ORIENTED_EDGE('',*,*,#16003,.F.);
#22168=ORIENTED_EDGE('',*,*,#16004,.F.);
#22169=ORIENTED_EDGE('',*,*,#16002,.F.);
#22170=ORIENTED_EDGE('',*,*,#16005,.F.);
#22171=ORIENTED_EDGE('',*,*,#16006,.F.);
#22172=ORIENTED_EDGE('',*,*,#16007,.F.);
#22173=ORIENTED_EDGE('',*,*,#16005,.T.);
#22174=ORIENTED_EDGE('',*,*,#16001,.F.);
#22175=ORIENTED_EDGE('',*,*,#16008,.F.);
#22176=ORIENTED_EDGE('',*,*,#16009,.T.);
#22177=ORIENTED_EDGE('',*,*,#16010,.T.);
#22178=ORIENTED_EDGE('',*,*,#16011,.F.);
#22179=ORIENTED_EDGE('',*,*,#16012,.F.);
#22180=ORIENTED_EDGE('',*,*,#16010,.F.);
#22181=ORIENTED_EDGE('',*,*,#16013,.F.);
#22182=ORIENTED_EDGE('',*,*,#16014,.F.);
#22183=ORIENTED_EDGE('',*,*,#16015,.F.);
#22184=ORIENTED_EDGE('',*,*,#16013,.T.);
#22185=ORIENTED_EDGE('',*,*,#16009,.F.);
#22186=ORIENTED_EDGE('',*,*,#16016,.F.);
#22187=ORIENTED_EDGE('',*,*,#16017,.T.);
#22188=ORIENTED_EDGE('',*,*,#16018,.T.);
#22189=ORIENTED_EDGE('',*,*,#16019,.F.);
#22190=ORIENTED_EDGE('',*,*,#16020,.F.);
#22191=ORIENTED_EDGE('',*,*,#16018,.F.);
#22192=ORIENTED_EDGE('',*,*,#16021,.F.);
#22193=ORIENTED_EDGE('',*,*,#16022,.F.);
#22194=ORIENTED_EDGE('',*,*,#16023,.F.);
#22195=ORIENTED_EDGE('',*,*,#16021,.T.);
#22196=ORIENTED_EDGE('',*,*,#16017,.F.);
#22197=ORIENTED_EDGE('',*,*,#16024,.F.);
#22198=ORIENTED_EDGE('',*,*,#16025,.T.);
#22199=ORIENTED_EDGE('',*,*,#16026,.T.);
#22200=ORIENTED_EDGE('',*,*,#16027,.F.);
#22201=ORIENTED_EDGE('',*,*,#16028,.F.);
#22202=ORIENTED_EDGE('',*,*,#16026,.F.);
#22203=ORIENTED_EDGE('',*,*,#16029,.F.);
#22204=ORIENTED_EDGE('',*,*,#16030,.F.);
#22205=ORIENTED_EDGE('',*,*,#16031,.F.);
#22206=ORIENTED_EDGE('',*,*,#16029,.T.);
#22207=ORIENTED_EDGE('',*,*,#16025,.F.);
#22208=ORIENTED_EDGE('',*,*,#16032,.F.);
#22209=ORIENTED_EDGE('',*,*,#16033,.T.);
#22210=ORIENTED_EDGE('',*,*,#16034,.T.);
#22211=ORIENTED_EDGE('',*,*,#16035,.F.);
#22212=ORIENTED_EDGE('',*,*,#16036,.F.);
#22213=ORIENTED_EDGE('',*,*,#16034,.F.);
#22214=ORIENTED_EDGE('',*,*,#16037,.F.);
#22215=ORIENTED_EDGE('',*,*,#16038,.F.);
#22216=ORIENTED_EDGE('',*,*,#16039,.F.);
#22217=ORIENTED_EDGE('',*,*,#16037,.T.);
#22218=ORIENTED_EDGE('',*,*,#16033,.F.);
#22219=ORIENTED_EDGE('',*,*,#16040,.F.);
#22220=ORIENTED_EDGE('',*,*,#16041,.T.);
#22221=ORIENTED_EDGE('',*,*,#16042,.T.);
#22222=ORIENTED_EDGE('',*,*,#16043,.F.);
#22223=ORIENTED_EDGE('',*,*,#16044,.F.);
#22224=ORIENTED_EDGE('',*,*,#16042,.F.);
#22225=ORIENTED_EDGE('',*,*,#16045,.F.);
#22226=ORIENTED_EDGE('',*,*,#16046,.F.);
#22227=ORIENTED_EDGE('',*,*,#16047,.F.);
#22228=ORIENTED_EDGE('',*,*,#16045,.T.);
#22229=ORIENTED_EDGE('',*,*,#16041,.F.);
#22230=ORIENTED_EDGE('',*,*,#16048,.F.);
#22231=ORIENTED_EDGE('',*,*,#16049,.T.);
#22232=ORIENTED_EDGE('',*,*,#16050,.T.);
#22233=ORIENTED_EDGE('',*,*,#16051,.F.);
#22234=ORIENTED_EDGE('',*,*,#16052,.F.);
#22235=ORIENTED_EDGE('',*,*,#16050,.F.);
#22236=ORIENTED_EDGE('',*,*,#16053,.F.);
#22237=ORIENTED_EDGE('',*,*,#16054,.F.);
#22238=ORIENTED_EDGE('',*,*,#16055,.F.);
#22239=ORIENTED_EDGE('',*,*,#16053,.T.);
#22240=ORIENTED_EDGE('',*,*,#16049,.F.);
#22241=ORIENTED_EDGE('',*,*,#16056,.F.);
#22242=ORIENTED_EDGE('',*,*,#16057,.T.);
#22243=ORIENTED_EDGE('',*,*,#16058,.T.);
#22244=ORIENTED_EDGE('',*,*,#16059,.F.);
#22245=ORIENTED_EDGE('',*,*,#16060,.F.);
#22246=ORIENTED_EDGE('',*,*,#16058,.F.);
#22247=ORIENTED_EDGE('',*,*,#16061,.F.);
#22248=ORIENTED_EDGE('',*,*,#16062,.F.);
#22249=ORIENTED_EDGE('',*,*,#16063,.F.);
#22250=ORIENTED_EDGE('',*,*,#16061,.T.);
#22251=ORIENTED_EDGE('',*,*,#16057,.F.);
#22252=ORIENTED_EDGE('',*,*,#16064,.F.);
#22253=ORIENTED_EDGE('',*,*,#16065,.T.);
#22254=ORIENTED_EDGE('',*,*,#16066,.T.);
#22255=ORIENTED_EDGE('',*,*,#16067,.F.);
#22256=ORIENTED_EDGE('',*,*,#16068,.F.);
#22257=ORIENTED_EDGE('',*,*,#16066,.F.);
#22258=ORIENTED_EDGE('',*,*,#16069,.F.);
#22259=ORIENTED_EDGE('',*,*,#16070,.F.);
#22260=ORIENTED_EDGE('',*,*,#16071,.F.);
#22261=ORIENTED_EDGE('',*,*,#16069,.T.);
#22262=ORIENTED_EDGE('',*,*,#16065,.F.);
#22263=ORIENTED_EDGE('',*,*,#16072,.F.);
#22264=ORIENTED_EDGE('',*,*,#16073,.T.);
#22265=ORIENTED_EDGE('',*,*,#16074,.T.);
#22266=ORIENTED_EDGE('',*,*,#16075,.F.);
#22267=ORIENTED_EDGE('',*,*,#16076,.F.);
#22268=ORIENTED_EDGE('',*,*,#16074,.F.);
#22269=ORIENTED_EDGE('',*,*,#16077,.F.);
#22270=ORIENTED_EDGE('',*,*,#16078,.F.);
#22271=ORIENTED_EDGE('',*,*,#16079,.F.);
#22272=ORIENTED_EDGE('',*,*,#16077,.T.);
#22273=ORIENTED_EDGE('',*,*,#16073,.F.);
#22274=ORIENTED_EDGE('',*,*,#16080,.F.);
#22275=ORIENTED_EDGE('',*,*,#16081,.T.);
#22276=ORIENTED_EDGE('',*,*,#16082,.T.);
#22277=ORIENTED_EDGE('',*,*,#16083,.F.);
#22278=ORIENTED_EDGE('',*,*,#16084,.F.);
#22279=ORIENTED_EDGE('',*,*,#16082,.F.);
#22280=ORIENTED_EDGE('',*,*,#16085,.F.);
#22281=ORIENTED_EDGE('',*,*,#16086,.F.);
#22282=ORIENTED_EDGE('',*,*,#16087,.F.);
#22283=ORIENTED_EDGE('',*,*,#16085,.T.);
#22284=ORIENTED_EDGE('',*,*,#16081,.F.);
#22285=ORIENTED_EDGE('',*,*,#16088,.F.);
#22286=ORIENTED_EDGE('',*,*,#16089,.T.);
#22287=ORIENTED_EDGE('',*,*,#16090,.T.);
#22288=ORIENTED_EDGE('',*,*,#16091,.F.);
#22289=ORIENTED_EDGE('',*,*,#16092,.F.);
#22290=ORIENTED_EDGE('',*,*,#16090,.F.);
#22291=ORIENTED_EDGE('',*,*,#16093,.F.);
#22292=ORIENTED_EDGE('',*,*,#16094,.F.);
#22293=ORIENTED_EDGE('',*,*,#16095,.F.);
#22294=ORIENTED_EDGE('',*,*,#16093,.T.);
#22295=ORIENTED_EDGE('',*,*,#16089,.F.);
#22296=ORIENTED_EDGE('',*,*,#16096,.F.);
#22297=ORIENTED_EDGE('',*,*,#16097,.T.);
#22298=ORIENTED_EDGE('',*,*,#16098,.T.);
#22299=ORIENTED_EDGE('',*,*,#16099,.F.);
#22300=ORIENTED_EDGE('',*,*,#16100,.F.);
#22301=ORIENTED_EDGE('',*,*,#16098,.F.);
#22302=ORIENTED_EDGE('',*,*,#16101,.F.);
#22303=ORIENTED_EDGE('',*,*,#16102,.F.);
#22304=ORIENTED_EDGE('',*,*,#16103,.F.);
#22305=ORIENTED_EDGE('',*,*,#16104,.F.);
#22306=ORIENTED_EDGE('',*,*,#16101,.T.);
#22307=ORIENTED_EDGE('',*,*,#16097,.F.);
#22308=ORIENTED_EDGE('',*,*,#16105,.F.);
#22309=ORIENTED_EDGE('',*,*,#16106,.T.);
#22310=ORIENTED_EDGE('',*,*,#16107,.T.);
#22311=ORIENTED_EDGE('',*,*,#16108,.F.);
#22312=ORIENTED_EDGE('',*,*,#16109,.F.);
#22313=ORIENTED_EDGE('',*,*,#16107,.F.);
#22314=ORIENTED_EDGE('',*,*,#16110,.F.);
#22315=ORIENTED_EDGE('',*,*,#16111,.F.);
#22316=ORIENTED_EDGE('',*,*,#16112,.F.);
#22317=ORIENTED_EDGE('',*,*,#16110,.T.);
#22318=ORIENTED_EDGE('',*,*,#16106,.F.);
#22319=ORIENTED_EDGE('',*,*,#16113,.F.);
#22320=ORIENTED_EDGE('',*,*,#16114,.T.);
#22321=ORIENTED_EDGE('',*,*,#16115,.T.);
#22322=ORIENTED_EDGE('',*,*,#16116,.F.);
#22323=ORIENTED_EDGE('',*,*,#16117,.F.);
#22324=ORIENTED_EDGE('',*,*,#16115,.F.);
#22325=ORIENTED_EDGE('',*,*,#16118,.F.);
#22326=ORIENTED_EDGE('',*,*,#16119,.F.);
#22327=ORIENTED_EDGE('',*,*,#16120,.F.);
#22328=ORIENTED_EDGE('',*,*,#16118,.T.);
#22329=ORIENTED_EDGE('',*,*,#16114,.F.);
#22330=ORIENTED_EDGE('',*,*,#16121,.F.);
#22331=ORIENTED_EDGE('',*,*,#16122,.T.);
#22332=ORIENTED_EDGE('',*,*,#16123,.T.);
#22333=ORIENTED_EDGE('',*,*,#16124,.F.);
#22334=ORIENTED_EDGE('',*,*,#16125,.F.);
#22335=ORIENTED_EDGE('',*,*,#16123,.F.);
#22336=ORIENTED_EDGE('',*,*,#16126,.F.);
#22337=ORIENTED_EDGE('',*,*,#16127,.F.);
#22338=ORIENTED_EDGE('',*,*,#16128,.F.);
#22339=ORIENTED_EDGE('',*,*,#16126,.T.);
#22340=ORIENTED_EDGE('',*,*,#16122,.F.);
#22341=ORIENTED_EDGE('',*,*,#16129,.F.);
#22342=ORIENTED_EDGE('',*,*,#16130,.T.);
#22343=ORIENTED_EDGE('',*,*,#16131,.T.);
#22344=ORIENTED_EDGE('',*,*,#16132,.F.);
#22345=ORIENTED_EDGE('',*,*,#16133,.F.);
#22346=ORIENTED_EDGE('',*,*,#16131,.F.);
#22347=ORIENTED_EDGE('',*,*,#16134,.F.);
#22348=ORIENTED_EDGE('',*,*,#16135,.F.);
#22349=ORIENTED_EDGE('',*,*,#16136,.F.);
#22350=ORIENTED_EDGE('',*,*,#16134,.T.);
#22351=ORIENTED_EDGE('',*,*,#16130,.F.);
#22352=ORIENTED_EDGE('',*,*,#15995,.T.);
#22353=ORIENTED_EDGE('',*,*,#15996,.T.);
#22354=ORIENTED_EDGE('',*,*,#15999,.T.);
#22355=ORIENTED_EDGE('',*,*,#16137,.F.);
#22356=ORIENTED_EDGE('',*,*,#16124,.T.);
#22357=ORIENTED_EDGE('',*,*,#16125,.T.);
#22358=ORIENTED_EDGE('',*,*,#16128,.T.);
#22359=ORIENTED_EDGE('',*,*,#16138,.F.);
#22360=ORIENTED_EDGE('',*,*,#16003,.T.);
#22361=ORIENTED_EDGE('',*,*,#16004,.T.);
#22362=ORIENTED_EDGE('',*,*,#16007,.T.);
#22363=ORIENTED_EDGE('',*,*,#16139,.F.);
#22364=ORIENTED_EDGE('',*,*,#16116,.T.);
#22365=ORIENTED_EDGE('',*,*,#16117,.T.);
#22366=ORIENTED_EDGE('',*,*,#16120,.T.);
#22367=ORIENTED_EDGE('',*,*,#16140,.F.);
#22368=ORIENTED_EDGE('',*,*,#16011,.T.);
#22369=ORIENTED_EDGE('',*,*,#16012,.T.);
#22370=ORIENTED_EDGE('',*,*,#16015,.T.);
#22371=ORIENTED_EDGE('',*,*,#16141,.F.);
#22372=ORIENTED_EDGE('',*,*,#16108,.T.);
#22373=ORIENTED_EDGE('',*,*,#16109,.T.);
#22374=ORIENTED_EDGE('',*,*,#16112,.T.);
#22375=ORIENTED_EDGE('',*,*,#16142,.F.);
#22376=ORIENTED_EDGE('',*,*,#16019,.T.);
#22377=ORIENTED_EDGE('',*,*,#16020,.T.);
#22378=ORIENTED_EDGE('',*,*,#16023,.T.);
#22379=ORIENTED_EDGE('',*,*,#16143,.F.);
#22380=ORIENTED_EDGE('',*,*,#16099,.T.);
#22381=ORIENTED_EDGE('',*,*,#16100,.T.);
#22382=ORIENTED_EDGE('',*,*,#16144,.T.);
#22383=ORIENTED_EDGE('',*,*,#16145,.T.);
#22384=ORIENTED_EDGE('',*,*,#16144,.F.);
#22385=ORIENTED_EDGE('',*,*,#16102,.T.);
#22386=ORIENTED_EDGE('',*,*,#16104,.T.);
#22387=ORIENTED_EDGE('',*,*,#16146,.F.);
#22388=ORIENTED_EDGE('',*,*,#16091,.T.);
#22389=ORIENTED_EDGE('',*,*,#16092,.T.);
#22390=ORIENTED_EDGE('',*,*,#16095,.T.);
#22391=ORIENTED_EDGE('',*,*,#16147,.F.);
#22392=ORIENTED_EDGE('',*,*,#16035,.T.);
#22393=ORIENTED_EDGE('',*,*,#16036,.T.);
#22394=ORIENTED_EDGE('',*,*,#16039,.T.);
#22395=ORIENTED_EDGE('',*,*,#16148,.F.);
#22396=ORIENTED_EDGE('',*,*,#16083,.T.);
#22397=ORIENTED_EDGE('',*,*,#16084,.T.);
#22398=ORIENTED_EDGE('',*,*,#16087,.T.);
#22399=ORIENTED_EDGE('',*,*,#16149,.F.);
#22400=ORIENTED_EDGE('',*,*,#16043,.T.);
#22401=ORIENTED_EDGE('',*,*,#16044,.T.);
#22402=ORIENTED_EDGE('',*,*,#16047,.T.);
#22403=ORIENTED_EDGE('',*,*,#16150,.F.);
#22404=ORIENTED_EDGE('',*,*,#16075,.T.);
#22405=ORIENTED_EDGE('',*,*,#16076,.T.);
#22406=ORIENTED_EDGE('',*,*,#16079,.T.);
#22407=ORIENTED_EDGE('',*,*,#16151,.F.);
#22408=ORIENTED_EDGE('',*,*,#16051,.T.);
#22409=ORIENTED_EDGE('',*,*,#16052,.T.);
#22410=ORIENTED_EDGE('',*,*,#16055,.T.);
#22411=ORIENTED_EDGE('',*,*,#16152,.F.);
#22412=ORIENTED_EDGE('',*,*,#16067,.T.);
#22413=ORIENTED_EDGE('',*,*,#16068,.T.);
#22414=ORIENTED_EDGE('',*,*,#16071,.T.);
#22415=ORIENTED_EDGE('',*,*,#16153,.F.);
#22416=ORIENTED_EDGE('',*,*,#16059,.T.);
#22417=ORIENTED_EDGE('',*,*,#16060,.T.);
#22418=ORIENTED_EDGE('',*,*,#16063,.T.);
#22419=ORIENTED_EDGE('',*,*,#16154,.F.);
#22420=ORIENTED_EDGE('',*,*,#16027,.T.);
#22421=ORIENTED_EDGE('',*,*,#16028,.T.);
#22422=ORIENTED_EDGE('',*,*,#16031,.T.);
#22423=ORIENTED_EDGE('',*,*,#16155,.F.);
#22424=ORIENTED_EDGE('',*,*,#16132,.T.);
#22425=ORIENTED_EDGE('',*,*,#16133,.T.);
#22426=ORIENTED_EDGE('',*,*,#16136,.T.);
#22427=ORIENTED_EDGE('',*,*,#16156,.F.);
#22428=ORIENTED_EDGE('',*,*,#16157,.F.);
#22429=ORIENTED_EDGE('',*,*,#16158,.F.);
#22430=ORIENTED_EDGE('',*,*,#15945,.F.);
#22431=ORIENTED_EDGE('',*,*,#15942,.F.);
#22432=ORIENTED_EDGE('',*,*,#15939,.F.);
#22433=ORIENTED_EDGE('',*,*,#15936,.F.);
#22434=ORIENTED_EDGE('',*,*,#15933,.F.);
#22435=ORIENTED_EDGE('',*,*,#15930,.F.);
#22436=ORIENTED_EDGE('',*,*,#15927,.F.);
#22437=ORIENTED_EDGE('',*,*,#15924,.F.);
#22438=ORIENTED_EDGE('',*,*,#15921,.F.);
#22439=ORIENTED_EDGE('',*,*,#15918,.F.);
#22440=ORIENTED_EDGE('',*,*,#15915,.F.);
#22441=ORIENTED_EDGE('',*,*,#15912,.F.);
#22442=ORIENTED_EDGE('',*,*,#15909,.F.);
#22443=ORIENTED_EDGE('',*,*,#15906,.F.);
#22444=ORIENTED_EDGE('',*,*,#15903,.F.);
#22445=ORIENTED_EDGE('',*,*,#16159,.F.);
#22446=ORIENTED_EDGE('',*,*,#16160,.T.);
#22447=ORIENTED_EDGE('',*,*,#15991,.T.);
#22448=ORIENTED_EDGE('',*,*,#15988,.T.);
#22449=ORIENTED_EDGE('',*,*,#15985,.T.);
#22450=ORIENTED_EDGE('',*,*,#15982,.T.);
#22451=ORIENTED_EDGE('',*,*,#15979,.T.);
#22452=ORIENTED_EDGE('',*,*,#15976,.T.);
#22453=ORIENTED_EDGE('',*,*,#15973,.T.);
#22454=ORIENTED_EDGE('',*,*,#15970,.T.);
#22455=ORIENTED_EDGE('',*,*,#15967,.T.);
#22456=ORIENTED_EDGE('',*,*,#15964,.T.);
#22457=ORIENTED_EDGE('',*,*,#15961,.T.);
#22458=ORIENTED_EDGE('',*,*,#15958,.T.);
#22459=ORIENTED_EDGE('',*,*,#15955,.T.);
#22460=ORIENTED_EDGE('',*,*,#15952,.T.);
#22461=ORIENTED_EDGE('',*,*,#15949,.T.);
#22462=ORIENTED_EDGE('',*,*,#16161,.T.);
#22463=ORIENTED_EDGE('',*,*,#16162,.T.);
#22464=ORIENTED_EDGE('',*,*,#16163,.T.);
#22465=ORIENTED_EDGE('',*,*,#16164,.T.);
#22466=ORIENTED_EDGE('',*,*,#16159,.T.);
#22467=ORIENTED_EDGE('',*,*,#15989,.T.);
#22468=ORIENTED_EDGE('',*,*,#16160,.F.);
#22469=ORIENTED_EDGE('',*,*,#16164,.F.);
#22470=ORIENTED_EDGE('',*,*,#16165,.T.);
#22471=ORIENTED_EDGE('',*,*,#16166,.F.);
#22472=ORIENTED_EDGE('',*,*,#15947,.F.);
#22473=ORIENTED_EDGE('',*,*,#15951,.F.);
#22474=ORIENTED_EDGE('',*,*,#15954,.F.);
#22475=ORIENTED_EDGE('',*,*,#15957,.F.);
#22476=ORIENTED_EDGE('',*,*,#15960,.F.);
#22477=ORIENTED_EDGE('',*,*,#15963,.F.);
#22478=ORIENTED_EDGE('',*,*,#15966,.F.);
#22479=ORIENTED_EDGE('',*,*,#15969,.F.);
#22480=ORIENTED_EDGE('',*,*,#15972,.F.);
#22481=ORIENTED_EDGE('',*,*,#15975,.F.);
#22482=ORIENTED_EDGE('',*,*,#15978,.F.);
#22483=ORIENTED_EDGE('',*,*,#15981,.F.);
#22484=ORIENTED_EDGE('',*,*,#15984,.F.);
#22485=ORIENTED_EDGE('',*,*,#15987,.F.);
#22486=ORIENTED_EDGE('',*,*,#15990,.F.);
#22487=ORIENTED_EDGE('',*,*,#16165,.F.);
#22488=ORIENTED_EDGE('',*,*,#16163,.F.);
#22489=ORIENTED_EDGE('',*,*,#15901,.F.);
#22490=ORIENTED_EDGE('',*,*,#15905,.F.);
#22491=ORIENTED_EDGE('',*,*,#15908,.F.);
#22492=ORIENTED_EDGE('',*,*,#15911,.F.);
#22493=ORIENTED_EDGE('',*,*,#15914,.F.);
#22494=ORIENTED_EDGE('',*,*,#15917,.F.);
#22495=ORIENTED_EDGE('',*,*,#15920,.F.);
#22496=ORIENTED_EDGE('',*,*,#15923,.F.);
#22497=ORIENTED_EDGE('',*,*,#15926,.F.);
#22498=ORIENTED_EDGE('',*,*,#15929,.F.);
#22499=ORIENTED_EDGE('',*,*,#15932,.F.);
#22500=ORIENTED_EDGE('',*,*,#15935,.F.);
#22501=ORIENTED_EDGE('',*,*,#15938,.F.);
#22502=ORIENTED_EDGE('',*,*,#15941,.F.);
#22503=ORIENTED_EDGE('',*,*,#15944,.F.);
#22504=ORIENTED_EDGE('',*,*,#16167,.F.);
#22505=ORIENTED_EDGE('',*,*,#16168,.F.);
#22506=ORIENTED_EDGE('',*,*,#16161,.F.);
#22507=ORIENTED_EDGE('',*,*,#15902,.F.);
#22508=ORIENTED_EDGE('',*,*,#16162,.F.);
#22509=ORIENTED_EDGE('',*,*,#16169,.T.);
#22510=ORIENTED_EDGE('',*,*,#16168,.T.);
#22511=ORIENTED_EDGE('',*,*,#16169,.F.);
#22512=ORIENTED_EDGE('',*,*,#15943,.T.);
#22513=ORIENTED_EDGE('',*,*,#16158,.T.);
#22514=ORIENTED_EDGE('',*,*,#16170,.F.);
#22515=ORIENTED_EDGE('',*,*,#16167,.T.);
#22516=ORIENTED_EDGE('',*,*,#16171,.F.);
#22517=ORIENTED_EDGE('',*,*,#16170,.T.);
#22518=ORIENTED_EDGE('',*,*,#16157,.T.);
#22519=ORIENTED_EDGE('',*,*,#15948,.T.);
#22520=ORIENTED_EDGE('',*,*,#16166,.T.);
#22521=ORIENTED_EDGE('',*,*,#16145,.F.);
#22522=ORIENTED_EDGE('',*,*,#16172,.T.);
#22523=ORIENTED_EDGE('',*,*,#16171,.T.);
#22524=ORIENTED_EDGE('',*,*,#16172,.F.);
#22525=ORIENTED_EDGE('',*,*,#16173,.F.);
#22526=ORIENTED_EDGE('',*,*,#16174,.T.);
#22527=ORIENTED_EDGE('',*,*,#16096,.T.);
#22528=ORIENTED_EDGE('',*,*,#16143,.T.);
#22529=ORIENTED_EDGE('',*,*,#16022,.T.);
#22530=ORIENTED_EDGE('',*,*,#16016,.T.);
#22531=ORIENTED_EDGE('',*,*,#16142,.T.);
#22532=ORIENTED_EDGE('',*,*,#16111,.T.);
#22533=ORIENTED_EDGE('',*,*,#16105,.T.);
#22534=ORIENTED_EDGE('',*,*,#16141,.T.);
#22535=ORIENTED_EDGE('',*,*,#16014,.T.);
#22536=ORIENTED_EDGE('',*,*,#16008,.T.);
#22537=ORIENTED_EDGE('',*,*,#16140,.T.);
#22538=ORIENTED_EDGE('',*,*,#16119,.T.);
#22539=ORIENTED_EDGE('',*,*,#16113,.T.);
#22540=ORIENTED_EDGE('',*,*,#16139,.T.);
#22541=ORIENTED_EDGE('',*,*,#16006,.T.);
#22542=ORIENTED_EDGE('',*,*,#16000,.T.);
#22543=ORIENTED_EDGE('',*,*,#16138,.T.);
#22544=ORIENTED_EDGE('',*,*,#16127,.T.);
#22545=ORIENTED_EDGE('',*,*,#16121,.T.);
#22546=ORIENTED_EDGE('',*,*,#16137,.T.);
#22547=ORIENTED_EDGE('',*,*,#15998,.T.);
#22548=ORIENTED_EDGE('',*,*,#15992,.T.);
#22549=ORIENTED_EDGE('',*,*,#16156,.T.);
#22550=ORIENTED_EDGE('',*,*,#16135,.T.);
#22551=ORIENTED_EDGE('',*,*,#16129,.T.);
#22552=ORIENTED_EDGE('',*,*,#16155,.T.);
#22553=ORIENTED_EDGE('',*,*,#16030,.T.);
#22554=ORIENTED_EDGE('',*,*,#16024,.T.);
#22555=ORIENTED_EDGE('',*,*,#16154,.T.);
#22556=ORIENTED_EDGE('',*,*,#16062,.T.);
#22557=ORIENTED_EDGE('',*,*,#16056,.T.);
#22558=ORIENTED_EDGE('',*,*,#16153,.T.);
#22559=ORIENTED_EDGE('',*,*,#16070,.T.);
#22560=ORIENTED_EDGE('',*,*,#16064,.T.);
#22561=ORIENTED_EDGE('',*,*,#16152,.T.);
#22562=ORIENTED_EDGE('',*,*,#16054,.T.);
#22563=ORIENTED_EDGE('',*,*,#16048,.T.);
#22564=ORIENTED_EDGE('',*,*,#16151,.T.);
#22565=ORIENTED_EDGE('',*,*,#16078,.T.);
#22566=ORIENTED_EDGE('',*,*,#16072,.T.);
#22567=ORIENTED_EDGE('',*,*,#16150,.T.);
#22568=ORIENTED_EDGE('',*,*,#16046,.T.);
#22569=ORIENTED_EDGE('',*,*,#16040,.T.);
#22570=ORIENTED_EDGE('',*,*,#16149,.T.);
#22571=ORIENTED_EDGE('',*,*,#16086,.T.);
#22572=ORIENTED_EDGE('',*,*,#16080,.T.);
#22573=ORIENTED_EDGE('',*,*,#16148,.T.);
#22574=ORIENTED_EDGE('',*,*,#16038,.T.);
#22575=ORIENTED_EDGE('',*,*,#16032,.T.);
#22576=ORIENTED_EDGE('',*,*,#16147,.T.);
#22577=ORIENTED_EDGE('',*,*,#16094,.T.);
#22578=ORIENTED_EDGE('',*,*,#16088,.T.);
#22579=ORIENTED_EDGE('',*,*,#16146,.T.);
#22580=ORIENTED_EDGE('',*,*,#16103,.T.);
#22581=ORIENTED_EDGE('',*,*,#16174,.F.);
#22582=ORIENTED_EDGE('',*,*,#16173,.T.);
#26535=PLANE('',#29769);
#26536=PLANE('',#29770);
#26537=PLANE('',#29772);
#26538=PLANE('',#29773);
#26539=PLANE('',#29774);
#26540=PLANE('',#29776);
#26541=PLANE('',#29777);
#26542=PLANE('',#29778);
#26543=PLANE('',#29780);
#26544=PLANE('',#29781);
#26545=PLANE('',#29782);
#26546=PLANE('',#29784);
#26547=PLANE('',#29785);
#26548=PLANE('',#29786);
#26549=PLANE('',#29788);
#26550=PLANE('',#29789);
#26551=PLANE('',#29790);
#26552=PLANE('',#29792);
#26553=PLANE('',#29793);
#26554=PLANE('',#29794);
#26555=PLANE('',#29796);
#26556=PLANE('',#29797);
#26557=PLANE('',#29798);
#26558=PLANE('',#29800);
#26559=PLANE('',#29801);
#26560=PLANE('',#29802);
#26561=PLANE('',#29804);
#26562=PLANE('',#29805);
#26563=PLANE('',#29806);
#26564=PLANE('',#29808);
#26565=PLANE('',#29809);
#26566=PLANE('',#29810);
#26567=PLANE('',#29812);
#26568=PLANE('',#29813);
#26569=PLANE('',#29814);
#26570=PLANE('',#29816);
#26571=PLANE('',#29817);
#26572=PLANE('',#29818);
#26573=PLANE('',#29820);
#26574=PLANE('',#29821);
#26575=PLANE('',#29822);
#26576=PLANE('',#29825);
#26577=PLANE('',#29826);
#26578=PLANE('',#29827);
#26579=PLANE('',#29829);
#26580=PLANE('',#29830);
#26581=PLANE('',#29831);
#26582=PLANE('',#29833);
#26583=PLANE('',#29834);
#26584=PLANE('',#29835);
#26585=PLANE('',#29837);
#26586=PLANE('',#29838);
#26587=PLANE('',#29839);
#26588=PLANE('',#29841);
#26589=PLANE('',#29862);
#26590=PLANE('',#29867);
#26591=PLANE('',#29872);
#26592=PLANE('',#29877);
#27673=ADVANCED_FACE('',(#3765),#1628,.T.);
#27674=ADVANCED_FACE('',(#3766),#1629,.T.);
#27675=ADVANCED_FACE('',(#3767),#1630,.T.);
#27676=ADVANCED_FACE('',(#3768),#1631,.T.);
#27677=ADVANCED_FACE('',(#3769),#1632,.T.);
#27678=ADVANCED_FACE('',(#3770),#1633,.T.);
#27679=ADVANCED_FACE('',(#3771),#1634,.T.);
#27680=ADVANCED_FACE('',(#3772),#1635,.T.);
#27681=ADVANCED_FACE('',(#3773),#1636,.T.);
#27682=ADVANCED_FACE('',(#3774),#1637,.T.);
#27683=ADVANCED_FACE('',(#3775),#1638,.T.);
#27684=ADVANCED_FACE('',(#3776),#1639,.T.);
#27685=ADVANCED_FACE('',(#3777),#1640,.T.);
#27686=ADVANCED_FACE('',(#3778),#1641,.T.);
#27687=ADVANCED_FACE('',(#3779),#1642,.T.);
#27688=ADVANCED_FACE('',(#3780),#1643,.T.);
#27689=ADVANCED_FACE('',(#3781),#1644,.T.);
#27690=ADVANCED_FACE('',(#3782),#1645,.T.);
#27691=ADVANCED_FACE('',(#3783),#1646,.T.);
#27692=ADVANCED_FACE('',(#3784),#1647,.T.);
#27693=ADVANCED_FACE('',(#3785),#1648,.T.);
#27694=ADVANCED_FACE('',(#3786),#1649,.T.);
#27695=ADVANCED_FACE('',(#3787),#1650,.T.);
#27696=ADVANCED_FACE('',(#3788),#1651,.T.);
#27697=ADVANCED_FACE('',(#3789),#1652,.T.);
#27698=ADVANCED_FACE('',(#3790),#1653,.T.);
#27699=ADVANCED_FACE('',(#3791),#1654,.T.);
#27700=ADVANCED_FACE('',(#3792),#1655,.T.);
#27701=ADVANCED_FACE('',(#3793),#1656,.T.);
#27702=ADVANCED_FACE('',(#3794),#1657,.T.);
#27703=ADVANCED_FACE('',(#3795),#26535,.F.);
#27704=ADVANCED_FACE('',(#3796),#26536,.F.);
#27705=ADVANCED_FACE('',(#3797),#26537,.F.);
#27706=ADVANCED_FACE('',(#3798),#26538,.F.);
#27707=ADVANCED_FACE('',(#3799),#26539,.F.);
#27708=ADVANCED_FACE('',(#3800),#26540,.F.);
#27709=ADVANCED_FACE('',(#3801),#26541,.F.);
#27710=ADVANCED_FACE('',(#3802),#26542,.F.);
#27711=ADVANCED_FACE('',(#3803),#26543,.F.);
#27712=ADVANCED_FACE('',(#3804),#26544,.F.);
#27713=ADVANCED_FACE('',(#3805),#26545,.F.);
#27714=ADVANCED_FACE('',(#3806),#26546,.F.);
#27715=ADVANCED_FACE('',(#3807),#26547,.F.);
#27716=ADVANCED_FACE('',(#3808),#26548,.F.);
#27717=ADVANCED_FACE('',(#3809),#26549,.F.);
#27718=ADVANCED_FACE('',(#3810),#26550,.F.);
#27719=ADVANCED_FACE('',(#3811),#26551,.F.);
#27720=ADVANCED_FACE('',(#3812),#26552,.F.);
#27721=ADVANCED_FACE('',(#3813),#26553,.F.);
#27722=ADVANCED_FACE('',(#3814),#26554,.F.);
#27723=ADVANCED_FACE('',(#3815),#26555,.F.);
#27724=ADVANCED_FACE('',(#3816),#26556,.F.);
#27725=ADVANCED_FACE('',(#3817),#26557,.F.);
#27726=ADVANCED_FACE('',(#3818),#26558,.F.);
#27727=ADVANCED_FACE('',(#3819),#26559,.F.);
#27728=ADVANCED_FACE('',(#3820),#26560,.F.);
#27729=ADVANCED_FACE('',(#3821),#26561,.F.);
#27730=ADVANCED_FACE('',(#3822),#26562,.F.);
#27731=ADVANCED_FACE('',(#3823),#26563,.F.);
#27732=ADVANCED_FACE('',(#3824),#26564,.F.);
#27733=ADVANCED_FACE('',(#3825),#26565,.F.);
#27734=ADVANCED_FACE('',(#3826),#26566,.F.);
#27735=ADVANCED_FACE('',(#3827),#26567,.F.);
#27736=ADVANCED_FACE('',(#3828),#26568,.F.);
#27737=ADVANCED_FACE('',(#3829),#26569,.F.);
#27738=ADVANCED_FACE('',(#3830),#26570,.F.);
#27739=ADVANCED_FACE('',(#3831),#26571,.F.);
#27740=ADVANCED_FACE('',(#3832),#26572,.F.);
#27741=ADVANCED_FACE('',(#3833),#26573,.F.);
#27742=ADVANCED_FACE('',(#3834),#26574,.F.);
#27743=ADVANCED_FACE('',(#3835),#26575,.F.);
#27744=ADVANCED_FACE('',(#3836),#26576,.F.);
#27745=ADVANCED_FACE('',(#3837),#26577,.F.);
#27746=ADVANCED_FACE('',(#3838),#26578,.F.);
#27747=ADVANCED_FACE('',(#3839),#26579,.F.);
#27748=ADVANCED_FACE('',(#3840),#26580,.F.);
#27749=ADVANCED_FACE('',(#3841),#26581,.F.);
#27750=ADVANCED_FACE('',(#3842),#26582,.F.);
#27751=ADVANCED_FACE('',(#3843),#26583,.F.);
#27752=ADVANCED_FACE('',(#3844),#26584,.F.);
#27753=ADVANCED_FACE('',(#3845),#26585,.F.);
#27754=ADVANCED_FACE('',(#3846),#26586,.F.);
#27755=ADVANCED_FACE('',(#3847),#26587,.F.);
#27756=ADVANCED_FACE('',(#3848),#26588,.F.);
#27757=ADVANCED_FACE('',(#3849),#1658,.T.);
#27758=ADVANCED_FACE('',(#3850),#1456,.F.);
#27759=ADVANCED_FACE('',(#3851),#26589,.F.);
#27760=ADVANCED_FACE('',(#3852),#1659,.T.);
#27761=ADVANCED_FACE('',(#3853),#1457,.F.);
#27762=ADVANCED_FACE('',(#3854),#26590,.T.);
#27763=ADVANCED_FACE('',(#3855),#2856,.T.);
#27764=ADVANCED_FACE('',(#3856),#1660,.T.);
#27765=ADVANCED_FACE('',(#3857,#1930),#26591,.T.);
#27766=ADVANCED_FACE('',(#3858),#2857,.T.);
#27767=ADVANCED_FACE('',(#3859),#2858,.T.);
#27768=ADVANCED_FACE('',(#3860),#26592,.T.);
#28465=CLOSED_SHELL('',(#27673,#27674,#27675,#27676,#27677,#27678,#27679,
#27680,#27681,#27682,#27683,#27684,#27685,#27686,#27687,#27688,#27689,#27690,
#27691,#27692,#27693,#27694,#27695,#27696,#27697,#27698,#27699,#27700,#27701,
#27702,#27703,#27704,#27705,#27706,#27707,#27708,#27709,#27710,#27711,#27712,
#27713,#27714,#27715,#27716,#27717,#27718,#27719,#27720,#27721,#27722,#27723,
#27724,#27725,#27726,#27727,#27728,#27729,#27730,#27731,#27732,#27733,#27734,
#27735,#27736,#27737,#27738,#27739,#27740,#27741,#27742,#27743,#27744,#27745,
#27746,#27747,#27748,#27749,#27750,#27751,#27752,#27753,#27754,#27755,#27756,
#27757,#27758,#27759,#27760,#27761,#27762,#27763,#27764,#27765,#27766,#27767,
#27768));
#29736=AXIS2_PLACEMENT_3D('',#46066,#34346,#34347);
#29737=AXIS2_PLACEMENT_3D('',#46067,#34348,#34349);
#29738=AXIS2_PLACEMENT_3D('',#46083,#34351,#34352);
#29739=AXIS2_PLACEMENT_3D('',#46094,#34353,#34354);
#29740=AXIS2_PLACEMENT_3D('',#46142,#34356,#34357);
#29741=AXIS2_PLACEMENT_3D('',#46190,#34359,#34360);
#29742=AXIS2_PLACEMENT_3D('',#46244,#34362,#34363);
#29743=AXIS2_PLACEMENT_3D('',#46292,#34365,#34366);
#29744=AXIS2_PLACEMENT_3D('',#46340,#34368,#34369);
#29745=AXIS2_PLACEMENT_3D('',#46394,#34371,#34372);
#29746=AXIS2_PLACEMENT_3D('',#46442,#34374,#34375);
#29747=AXIS2_PLACEMENT_3D('',#46490,#34377,#34378);
#29748=AXIS2_PLACEMENT_3D('',#46544,#34380,#34381);
#29749=AXIS2_PLACEMENT_3D('',#46592,#34383,#34384);
#29750=AXIS2_PLACEMENT_3D('',#46640,#34386,#34387);
#29751=AXIS2_PLACEMENT_3D('',#46688,#34389,#34390);
#29752=AXIS2_PLACEMENT_3D('',#46736,#34392,#34393);
#29753=AXIS2_PLACEMENT_3D('',#46784,#34395,#34396);
#29754=AXIS2_PLACEMENT_3D('',#46795,#34398,#34399);
#29755=AXIS2_PLACEMENT_3D('',#46800,#34400,#34401);
#29756=AXIS2_PLACEMENT_3D('',#46825,#34403,#34404);
#29757=AXIS2_PLACEMENT_3D('',#46849,#34406,#34407);
#29758=AXIS2_PLACEMENT_3D('',#46875,#34409,#34410);
#29759=AXIS2_PLACEMENT_3D('',#46899,#34412,#34413);
#29760=AXIS2_PLACEMENT_3D('',#46923,#34415,#34416);
#29761=AXIS2_PLACEMENT_3D('',#46948,#34418,#34419);
#29762=AXIS2_PLACEMENT_3D('',#46973,#34421,#34422);
#29763=AXIS2_PLACEMENT_3D('',#46997,#34424,#34425);
#29764=AXIS2_PLACEMENT_3D('',#47022,#34427,#34428);
#29765=AXIS2_PLACEMENT_3D('',#47047,#34430,#34431);
#29766=AXIS2_PLACEMENT_3D('',#47071,#34433,#34434);
#29767=AXIS2_PLACEMENT_3D('',#47096,#34436,#34437);
#29768=AXIS2_PLACEMENT_3D('',#47121,#34439,#34440);
#29769=AXIS2_PLACEMENT_3D('',#47145,#34442,#34443);
#29770=AXIS2_PLACEMENT_3D('',#47156,#34447,#34448);
#29771=AXIS2_PLACEMENT_3D('',#47158,#34449,#34450);
#29772=AXIS2_PLACEMENT_3D('',#47160,#34452,#34453);
#29773=AXIS2_PLACEMENT_3D('',#47166,#34455,#34456);
#29774=AXIS2_PLACEMENT_3D('',#47177,#34460,#34461);
#29775=AXIS2_PLACEMENT_3D('',#47179,#34462,#34463);
#29776=AXIS2_PLACEMENT_3D('',#47181,#34465,#34466);
#29777=AXIS2_PLACEMENT_3D('',#47187,#34468,#34469);
#29778=AXIS2_PLACEMENT_3D('',#47198,#34473,#34474);
#29779=AXIS2_PLACEMENT_3D('',#47200,#34475,#34476);
#29780=AXIS2_PLACEMENT_3D('',#47202,#34478,#34479);
#29781=AXIS2_PLACEMENT_3D('',#47208,#34481,#34482);
#29782=AXIS2_PLACEMENT_3D('',#47219,#34486,#34487);
#29783=AXIS2_PLACEMENT_3D('',#47221,#34488,#34489);
#29784=AXIS2_PLACEMENT_3D('',#47223,#34491,#34492);
#29785=AXIS2_PLACEMENT_3D('',#47229,#34494,#34495);
#29786=AXIS2_PLACEMENT_3D('',#47240,#34499,#34500);
#29787=AXIS2_PLACEMENT_3D('',#47242,#34501,#34502);
#29788=AXIS2_PLACEMENT_3D('',#47244,#34504,#34505);
#29789=AXIS2_PLACEMENT_3D('',#47250,#34507,#34508);
#29790=AXIS2_PLACEMENT_3D('',#47261,#34512,#34513);
#29791=AXIS2_PLACEMENT_3D('',#47263,#34514,#34515);
#29792=AXIS2_PLACEMENT_3D('',#47265,#34517,#34518);
#29793=AXIS2_PLACEMENT_3D('',#47271,#34520,#34521);
#29794=AXIS2_PLACEMENT_3D('',#47282,#34525,#34526);
#29795=AXIS2_PLACEMENT_3D('',#47284,#34527,#34528);
#29796=AXIS2_PLACEMENT_3D('',#47286,#34530,#34531);
#29797=AXIS2_PLACEMENT_3D('',#47292,#34533,#34534);
#29798=AXIS2_PLACEMENT_3D('',#47303,#34538,#34539);
#29799=AXIS2_PLACEMENT_3D('',#47305,#34540,#34541);
#29800=AXIS2_PLACEMENT_3D('',#47307,#34543,#34544);
#29801=AXIS2_PLACEMENT_3D('',#47313,#34546,#34547);
#29802=AXIS2_PLACEMENT_3D('',#47324,#34551,#34552);
#29803=AXIS2_PLACEMENT_3D('',#47326,#34553,#34554);
#29804=AXIS2_PLACEMENT_3D('',#47328,#34556,#34557);
#29805=AXIS2_PLACEMENT_3D('',#47334,#34559,#34560);
#29806=AXIS2_PLACEMENT_3D('',#47345,#34564,#34565);
#29807=AXIS2_PLACEMENT_3D('',#47347,#34566,#34567);
#29808=AXIS2_PLACEMENT_3D('',#47349,#34569,#34570);
#29809=AXIS2_PLACEMENT_3D('',#47355,#34572,#34573);
#29810=AXIS2_PLACEMENT_3D('',#47366,#34577,#34578);
#29811=AXIS2_PLACEMENT_3D('',#47368,#34579,#34580);
#29812=AXIS2_PLACEMENT_3D('',#47370,#34582,#34583);
#29813=AXIS2_PLACEMENT_3D('',#47376,#34585,#34586);
#29814=AXIS2_PLACEMENT_3D('',#47387,#34590,#34591);
#29815=AXIS2_PLACEMENT_3D('',#47389,#34592,#34593);
#29816=AXIS2_PLACEMENT_3D('',#47391,#34595,#34596);
#29817=AXIS2_PLACEMENT_3D('',#47397,#34598,#34599);
#29818=AXIS2_PLACEMENT_3D('',#47408,#34603,#34604);
#29819=AXIS2_PLACEMENT_3D('',#47410,#34605,#34606);
#29820=AXIS2_PLACEMENT_3D('',#47412,#34608,#34609);
#29821=AXIS2_PLACEMENT_3D('',#47418,#34611,#34612);
#29822=AXIS2_PLACEMENT_3D('',#47429,#34616,#34617);
#29823=AXIS2_PLACEMENT_3D('',#47431,#34618,#34619);
#29824=AXIS2_PLACEMENT_3D('',#47434,#34621,#34622);
#29825=AXIS2_PLACEMENT_3D('',#47435,#34623,#34624);
#29826=AXIS2_PLACEMENT_3D('',#47441,#34626,#34627);
#29827=AXIS2_PLACEMENT_3D('',#47452,#34631,#34632);
#29828=AXIS2_PLACEMENT_3D('',#47454,#34633,#34634);
#29829=AXIS2_PLACEMENT_3D('',#47456,#34636,#34637);
#29830=AXIS2_PLACEMENT_3D('',#47462,#34639,#34640);
#29831=AXIS2_PLACEMENT_3D('',#47473,#34644,#34645);
#29832=AXIS2_PLACEMENT_3D('',#47475,#34646,#34647);
#29833=AXIS2_PLACEMENT_3D('',#47477,#34649,#34650);
#29834=AXIS2_PLACEMENT_3D('',#47483,#34652,#34653);
#29835=AXIS2_PLACEMENT_3D('',#47494,#34657,#34658);
#29836=AXIS2_PLACEMENT_3D('',#47496,#34659,#34660);
#29837=AXIS2_PLACEMENT_3D('',#47498,#34662,#34663);
#29838=AXIS2_PLACEMENT_3D('',#47504,#34665,#34666);
#29839=AXIS2_PLACEMENT_3D('',#47515,#34670,#34671);
#29840=AXIS2_PLACEMENT_3D('',#47517,#34672,#34673);
#29841=AXIS2_PLACEMENT_3D('',#47519,#34675,#34676);
#29842=AXIS2_PLACEMENT_3D('',#47525,#34678,#34679);
#29843=AXIS2_PLACEMENT_3D('',#47526,#34680,#34681);
#29844=AXIS2_PLACEMENT_3D('',#47527,#34682,#34683);
#29845=AXIS2_PLACEMENT_3D('',#47528,#34684,#34685);
#29846=AXIS2_PLACEMENT_3D('',#47529,#34686,#34687);
#29847=AXIS2_PLACEMENT_3D('',#47530,#34688,#34689);
#29848=AXIS2_PLACEMENT_3D('',#47531,#34690,#34691);
#29849=AXIS2_PLACEMENT_3D('',#47532,#34692,#34693);
#29850=AXIS2_PLACEMENT_3D('',#47535,#34695,#34696);
#29851=AXIS2_PLACEMENT_3D('',#47536,#34697,#34698);
#29852=AXIS2_PLACEMENT_3D('',#47537,#34699,#34700);
#29853=AXIS2_PLACEMENT_3D('',#47538,#34701,#34702);
#29854=AXIS2_PLACEMENT_3D('',#47539,#34703,#34704);
#29855=AXIS2_PLACEMENT_3D('',#47540,#34705,#34706);
#29856=AXIS2_PLACEMENT_3D('',#47541,#34707,#34708);
#29857=AXIS2_PLACEMENT_3D('',#47542,#34709,#34710);
#29858=AXIS2_PLACEMENT_3D('',#47543,#34711,#34712);
#29859=AXIS2_PLACEMENT_3D('',#47544,#34713,#34714);
#29860=AXIS2_PLACEMENT_3D('',#47545,#34715,#34716);
#29861=AXIS2_PLACEMENT_3D('',#47546,#34717,#34718);
#29862=AXIS2_PLACEMENT_3D('',#48106,#34719,#34720);
#29863=AXIS2_PLACEMENT_3D('',#48108,#34721,#34722);
#29864=AXIS2_PLACEMENT_3D('',#48109,#34723,#34724);
#29865=AXIS2_PLACEMENT_3D('',#48175,#34725,#34726);
#29866=AXIS2_PLACEMENT_3D('',#48176,#34727,#34728);
#29867=AXIS2_PLACEMENT_3D('',#48671,#34729,#34730);
#29868=AXIS2_PLACEMENT_3D('',#48673,#34731,#34732);
#29869=AXIS2_PLACEMENT_3D('',#48674,#34733,#34734);
#29870=AXIS2_PLACEMENT_3D('',#48676,#34736,#34737);
#29871=AXIS2_PLACEMENT_3D('',#48677,#34738,#34739);
#29872=AXIS2_PLACEMENT_3D('',#48678,#34740,#34741);
#29873=AXIS2_PLACEMENT_3D('',#48680,#34742,#34743);
#29874=AXIS2_PLACEMENT_3D('',#48681,#34744,#34745);
#29875=AXIS2_PLACEMENT_3D('',#48683,#34747,#34748);
#29876=AXIS2_PLACEMENT_3D('',#48685,#34749,#34750);
#29877=AXIS2_PLACEMENT_3D('',#48687,#34752,#34753);
#34346=DIRECTION('axis',(0.,0.,1.));
#34347=DIRECTION('refdir',(1.,0.,0.));
#34348=DIRECTION('center_axis',(0.,-1.,0.));
#34349=DIRECTION('ref_axis',(1.,0.,0.));
#34350=DIRECTION('',(0.,1.,0.));
#34351=DIRECTION('center_axis',(0.,-1.,0.));
#34352=DIRECTION('ref_axis',(1.,0.,0.));
#34353=DIRECTION('center_axis',(0.,-1.,0.));
#34354=DIRECTION('ref_axis',(1.,0.,0.));
#34355=DIRECTION('',(0.,1.,0.));
#34356=DIRECTION('center_axis',(0.,-1.,0.));
#34357=DIRECTION('ref_axis',(1.,0.,0.));
#34358=DIRECTION('',(0.,1.,0.));
#34359=DIRECTION('center_axis',(0.,-1.,0.));
#34360=DIRECTION('ref_axis',(1.,0.,0.));
#34361=DIRECTION('',(0.,1.,0.));
#34362=DIRECTION('center_axis',(0.,-1.,0.));
#34363=DIRECTION('ref_axis',(1.,0.,0.));
#34364=DIRECTION('',(0.,1.,0.));
#34365=DIRECTION('center_axis',(0.,-1.,0.));
#34366=DIRECTION('ref_axis',(1.,0.,0.));
#34367=DIRECTION('',(0.,1.,0.));
#34368=DIRECTION('center_axis',(0.,-1.,0.));
#34369=DIRECTION('ref_axis',(1.,0.,0.));
#34370=DIRECTION('',(0.,1.,0.));
#34371=DIRECTION('center_axis',(0.,-1.,0.));
#34372=DIRECTION('ref_axis',(1.,0.,0.));
#34373=DIRECTION('',(0.,1.,0.));
#34374=DIRECTION('center_axis',(0.,-1.,0.));
#34375=DIRECTION('ref_axis',(1.,0.,0.));
#34376=DIRECTION('',(0.,1.,0.));
#34377=DIRECTION('center_axis',(0.,-1.,0.));
#34378=DIRECTION('ref_axis',(1.,0.,0.));
#34379=DIRECTION('',(0.,1.,0.));
#34380=DIRECTION('center_axis',(0.,-1.,0.));
#34381=DIRECTION('ref_axis',(1.,0.,0.));
#34382=DIRECTION('',(0.,1.,0.));
#34383=DIRECTION('center_axis',(0.,-1.,0.));
#34384=DIRECTION('ref_axis',(1.,0.,0.));
#34385=DIRECTION('',(0.,1.,0.));
#34386=DIRECTION('center_axis',(0.,-1.,0.));
#34387=DIRECTION('ref_axis',(1.,0.,0.));
#34388=DIRECTION('',(0.,1.,0.));
#34389=DIRECTION('center_axis',(0.,-1.,0.));
#34390=DIRECTION('ref_axis',(1.,0.,0.));
#34391=DIRECTION('',(0.,1.,0.));
#34392=DIRECTION('center_axis',(0.,-1.,0.));
#34393=DIRECTION('ref_axis',(1.,0.,0.));
#34394=DIRECTION('',(0.,1.,0.));
#34395=DIRECTION('center_axis',(0.,-1.,0.));
#34396=DIRECTION('ref_axis',(1.,0.,8.81908600741727E-14));
#34397=DIRECTION('',(0.,-1.,0.));
#34398=DIRECTION('center_axis',(0.,-1.,0.));
#34399=DIRECTION('ref_axis',(1.,0.,8.81908600741727E-14));
#34400=DIRECTION('center_axis',(0.,-1.,0.));
#34401=DIRECTION('ref_axis',(1.,0.,8.81908600741727E-14));
#34402=DIRECTION('',(0.,-1.,0.));
#34403=DIRECTION('center_axis',(0.,-1.,0.));
#34404=DIRECTION('ref_axis',(1.,0.,8.81908600741727E-14));
#34405=DIRECTION('',(0.,-1.,0.));
#34406=DIRECTION('center_axis',(0.,-1.,0.));
#34407=DIRECTION('ref_axis',(1.,0.,8.81908600741727E-14));
#34408=DIRECTION('',(0.,-1.,0.));
#34409=DIRECTION('center_axis',(0.,-1.,0.));
#34410=DIRECTION('ref_axis',(1.,0.,8.81908600741727E-14));
#34411=DIRECTION('',(0.,-1.,0.));
#34412=DIRECTION('center_axis',(0.,-1.,0.));
#34413=DIRECTION('ref_axis',(1.,0.,8.81908600741727E-14));
#34414=DIRECTION('',(0.,-1.,0.));
#34415=DIRECTION('center_axis',(0.,-1.,0.));
#34416=DIRECTION('ref_axis',(1.,0.,8.81908600741727E-14));
#34417=DIRECTION('',(0.,-1.,0.));
#34418=DIRECTION('center_axis',(0.,-1.,0.));
#34419=DIRECTION('ref_axis',(1.,0.,8.81908600741727E-14));
#34420=DIRECTION('',(0.,-1.,0.));
#34421=DIRECTION('center_axis',(0.,-1.,0.));
#34422=DIRECTION('ref_axis',(1.,0.,8.81908600741727E-14));
#34423=DIRECTION('',(0.,-1.,0.));
#34424=DIRECTION('center_axis',(0.,-1.,0.));
#34425=DIRECTION('ref_axis',(1.,0.,8.81908600741727E-14));
#34426=DIRECTION('',(0.,-1.,0.));
#34427=DIRECTION('center_axis',(0.,-1.,0.));
#34428=DIRECTION('ref_axis',(1.,0.,8.81908600741727E-14));
#34429=DIRECTION('',(0.,-1.,0.));
#34430=DIRECTION('center_axis',(0.,-1.,0.));
#34431=DIRECTION('ref_axis',(1.,0.,8.81908600741727E-14));
#34432=DIRECTION('',(0.,-1.,0.));
#34433=DIRECTION('center_axis',(0.,-1.,0.));
#34434=DIRECTION('ref_axis',(1.,0.,8.81908600741727E-14));
#34435=DIRECTION('',(0.,-1.,0.));
#34436=DIRECTION('center_axis',(0.,-1.,0.));
#34437=DIRECTION('ref_axis',(1.,0.,8.81908600741727E-14));
#34438=DIRECTION('',(0.,-1.,0.));
#34439=DIRECTION('center_axis',(0.,-1.,0.));
#34440=DIRECTION('ref_axis',(1.,0.,8.81908600741727E-14));
#34441=DIRECTION('',(0.,-1.,0.));
#34442=DIRECTION('center_axis',(-0.0386781209882463,0.,0.999251721518066));
#34443=DIRECTION('ref_axis',(0.999251721518066,0.,0.0386781209882463));
#34444=DIRECTION('',(0.,1.,0.));
#34445=DIRECTION('',(0.999251721518066,0.,0.0386781209882463));
#34446=DIRECTION('',(0.,1.,0.));
#34447=DIRECTION('center_axis',(0.,1.,0.));
#34448=DIRECTION('ref_axis',(0.,0.,1.));
#34449=DIRECTION('center_axis',(0.,1.,0.));
#34450=DIRECTION('ref_axis',(1.,0.,0.));
#34451=DIRECTION('',(-0.135427727050936,0.,0.990787227786984));
#34452=DIRECTION('center_axis',(-0.990787227786984,0.,-0.135427727050936));
#34453=DIRECTION('ref_axis',(-0.135427727050936,0.,0.990787227786984));
#34454=DIRECTION('',(0.,-1.,0.));
#34455=DIRECTION('center_axis',(0.612677465896384,0.,0.790333045483222));
#34456=DIRECTION('ref_axis',(0.790333045483222,0.,-0.612677465896384));
#34457=DIRECTION('',(0.,1.,0.));
#34458=DIRECTION('',(0.790333045483222,0.,-0.612677465896384));
#34459=DIRECTION('',(0.,1.,0.));
#34460=DIRECTION('center_axis',(0.,1.,0.));
#34461=DIRECTION('ref_axis',(0.,0.,1.));
#34462=DIRECTION('center_axis',(0.,1.,0.));
#34463=DIRECTION('ref_axis',(1.,0.,0.));
#34464=DIRECTION('',(0.53312209610552,0.,0.846038315115844));
#34465=DIRECTION('center_axis',(-0.846038315115844,0.,0.53312209610552));
#34466=DIRECTION('ref_axis',(0.53312209610552,0.,0.846038315115844));
#34467=DIRECTION('',(0.,-1.,0.));
#34468=DIRECTION('center_axis',(0.97735445733659,0.,0.211608753893357));
#34469=DIRECTION('ref_axis',(0.211608753893357,0.,-0.97735445733659));
#34470=DIRECTION('',(0.,1.,0.));
#34471=DIRECTION('',(0.211608753893357,0.,-0.97735445733659));
#34472=DIRECTION('',(0.,1.,0.));
#34473=DIRECTION('center_axis',(0.,1.,0.));
#34474=DIRECTION('ref_axis',(0.,0.,1.));
#34475=DIRECTION('center_axis',(0.,1.,0.));
#34476=DIRECTION('ref_axis',(1.,0.,0.));
#34477=DIRECTION('',(0.952218165502102,0.,0.305418672133534));
#34478=DIRECTION('center_axis',(-0.305418672133534,0.,0.952218165502102));
#34479=DIRECTION('ref_axis',(0.952218165502102,0.,0.305418672133534));
#34480=DIRECTION('',(0.,-1.,0.));
#34481=DIRECTION('center_axis',(0.884716436104133,0.,-0.466129625412504));
#34482=DIRECTION('ref_axis',(-0.466129625412504,0.,-0.884716436104133));
#34483=DIRECTION('',(0.,1.,0.));
#34484=DIRECTION('',(-0.466129625412504,0.,-0.884716436104133));
#34485=DIRECTION('',(0.,1.,0.));
#34486=DIRECTION('center_axis',(0.,1.,0.));
#34487=DIRECTION('ref_axis',(0.,0.,1.));
#34488=DIRECTION('center_axis',(0.,1.,0.));
#34489=DIRECTION('ref_axis',(1.,0.,0.));
#34490=DIRECTION('',(0.92576077253418,0.,-0.378109761890538));
#34491=DIRECTION('center_axis',(0.378109761890538,0.,0.92576077253418));
#34492=DIRECTION('ref_axis',(0.92576077253418,0.,-0.378109761890538));
#34493=DIRECTION('',(0.,-1.,0.));
#34494=DIRECTION('center_axis',(-0.671935785203098,0.,0.740609411608775));
#34495=DIRECTION('ref_axis',(0.740609411608775,0.,0.671935785203098));
#34496=DIRECTION('',(0.,1.,0.));
#34497=DIRECTION('',(0.740609411608775,0.,0.671935785203098));
#34498=DIRECTION('',(0.,1.,0.));
#34499=DIRECTION('center_axis',(0.,1.,0.));
#34500=DIRECTION('ref_axis',(0.,0.,1.));
#34501=DIRECTION('center_axis',(0.,1.,0.));
#34502=DIRECTION('ref_axis',(1.,0.,0.));
#34503=DIRECTION('',(-0.740609411608775,0.,0.671935785203098));
#34504=DIRECTION('center_axis',(-0.671935785203098,0.,-0.740609411608775));
#34505=DIRECTION('ref_axis',(-0.740609411608775,0.,0.671935785203098));
#34506=DIRECTION('',(0.,-1.,0.));
#34507=DIRECTION('center_axis',(0.0386781209882463,0.,-0.999251721518066));
#34508=DIRECTION('ref_axis',(-0.999251721518066,0.,-0.0386781209882463));
#34509=DIRECTION('',(0.,1.,0.));
#34510=DIRECTION('',(-0.999251721518066,0.,-0.0386781209882463));
#34511=DIRECTION('',(0.,1.,0.));
#34512=DIRECTION('center_axis',(0.,1.,0.));
#34513=DIRECTION('ref_axis',(0.,0.,1.));
#34514=DIRECTION('center_axis',(0.,1.,0.));
#34515=DIRECTION('ref_axis',(1.,0.,0.));
#34516=DIRECTION('',(0.135427727050939,0.,-0.990787227786984));
#34517=DIRECTION('center_axis',(0.990787227786984,0.,0.135427727050939));
#34518=DIRECTION('ref_axis',(0.135427727050939,0.,-0.990787227786984));
#34519=DIRECTION('',(0.,-1.,0.));
#34520=DIRECTION('center_axis',(-0.612677465896387,0.,-0.79033304548322));
#34521=DIRECTION('ref_axis',(-0.79033304548322,0.,0.612677465896387));
#34522=DIRECTION('',(0.,1.,0.));
#34523=DIRECTION('',(-0.79033304548322,0.,0.612677465896387));
#34524=DIRECTION('',(0.,1.,0.));
#34525=DIRECTION('center_axis',(0.,1.,0.));
#34526=DIRECTION('ref_axis',(0.,0.,1.));
#34527=DIRECTION('center_axis',(0.,1.,0.));
#34528=DIRECTION('ref_axis',(1.,0.,0.));
#34529=DIRECTION('',(-0.533122096105522,0.,-0.846038315115843));
#34530=DIRECTION('center_axis',(0.846038315115843,0.,-0.533122096105522));
#34531=DIRECTION('ref_axis',(-0.533122096105522,0.,-0.846038315115843));
#34532=DIRECTION('',(0.,-1.,0.));
#34533=DIRECTION('center_axis',(-0.977354457336591,0.,-0.211608753893355));
#34534=DIRECTION('ref_axis',(-0.211608753893355,0.,0.977354457336591));
#34535=DIRECTION('',(0.,1.,0.));
#34536=DIRECTION('',(-0.211608753893355,0.,0.977354457336591));
#34537=DIRECTION('',(0.,1.,0.));
#34538=DIRECTION('center_axis',(0.,1.,0.));
#34539=DIRECTION('ref_axis',(0.,0.,1.));
#34540=DIRECTION('center_axis',(0.,1.,0.));
#34541=DIRECTION('ref_axis',(1.,0.,0.));
#34542=DIRECTION('',(-0.952218165502102,0.,-0.305418672133534));
#34543=DIRECTION('center_axis',(0.305418672133534,0.,-0.952218165502102));
#34544=DIRECTION('ref_axis',(-0.952218165502102,0.,-0.305418672133534));
#34545=DIRECTION('',(0.,-1.,0.));
#34546=DIRECTION('center_axis',(-0.884716436104133,0.,0.466129625412504));
#34547=DIRECTION('ref_axis',(0.466129625412504,0.,0.884716436104133));
#34548=DIRECTION('',(0.,1.,0.));
#34549=DIRECTION('',(0.466129625412503,0.,0.884716436104133));
#34550=DIRECTION('',(0.,1.,0.));
#34551=DIRECTION('center_axis',(0.,1.,0.));
#34552=DIRECTION('ref_axis',(0.,0.,1.));
#34553=DIRECTION('center_axis',(0.,1.,0.));
#34554=DIRECTION('ref_axis',(1.,0.,0.));
#34555=DIRECTION('',(-0.925760772534179,0.,0.378109761890538));
#34556=DIRECTION('center_axis',(-0.378109761890538,0.,-0.925760772534179));
#34557=DIRECTION('ref_axis',(-0.925760772534179,0.,0.378109761890538));
#34558=DIRECTION('',(0.,-1.,0.));
#34559=DIRECTION('center_axis',(-0.990787227786984,0.,0.135427727050936));
#34560=DIRECTION('ref_axis',(0.135427727050936,0.,0.990787227786984));
#34561=DIRECTION('',(0.,1.,0.));
#34562=DIRECTION('',(0.135427727050936,0.,0.990787227786984));
#34563=DIRECTION('',(0.,1.,0.));
#34564=DIRECTION('center_axis',(0.,1.,0.));
#34565=DIRECTION('ref_axis',(0.,0.,1.));
#34566=DIRECTION('center_axis',(0.,1.,0.));
#34567=DIRECTION('ref_axis',(1.,0.,0.));
#34568=DIRECTION('',(-0.999251721518066,0.,0.0386781209882463));
#34569=DIRECTION('center_axis',(-0.0386781209882463,0.,-0.999251721518066));
#34570=DIRECTION('ref_axis',(-0.999251721518066,0.,0.0386781209882463));
#34571=DIRECTION('',(0.,-1.,0.));
#34572=DIRECTION('center_axis',(-0.846038315115843,0.,-0.533122096105522));
#34573=DIRECTION('ref_axis',(-0.533122096105522,0.,0.846038315115843));
#34574=DIRECTION('',(0.,1.,0.));
#34575=DIRECTION('',(-0.533122096105522,0.,0.846038315115843));
#34576=DIRECTION('',(0.,1.,0.));
#34577=DIRECTION('center_axis',(0.,1.,0.));
#34578=DIRECTION('ref_axis',(0.,0.,1.));
#34579=DIRECTION('center_axis',(0.,1.,0.));
#34580=DIRECTION('ref_axis',(1.,0.,0.));
#34581=DIRECTION('',(-0.790333045483219,0.,-0.612677465896388));
#34582=DIRECTION('center_axis',(0.612677465896388,0.,-0.790333045483219));
#34583=DIRECTION('ref_axis',(-0.790333045483219,0.,-0.612677465896388));
#34584=DIRECTION('',(0.,-1.,0.));
#34585=DIRECTION('center_axis',(-0.305418672133533,0.,-0.952218165502102));
#34586=DIRECTION('ref_axis',(-0.952218165502102,0.,0.305418672133533));
#34587=DIRECTION('',(0.,1.,0.));
#34588=DIRECTION('',(-0.952218165502102,0.,0.305418672133533));
#34589=DIRECTION('',(0.,1.,0.));
#34590=DIRECTION('center_axis',(0.,1.,0.));
#34591=DIRECTION('ref_axis',(0.,0.,1.));
#34592=DIRECTION('center_axis',(0.,1.,0.));
#34593=DIRECTION('ref_axis',(1.,0.,0.));
#34594=DIRECTION('',(-0.211608753893352,0.,-0.977354457336591));
#34595=DIRECTION('center_axis',(0.977354457336591,0.,-0.211608753893352));
#34596=DIRECTION('ref_axis',(-0.211608753893352,0.,-0.977354457336591));
#34597=DIRECTION('',(0.,-1.,0.));
#34598=DIRECTION('center_axis',(0.378109761890538,0.,-0.92576077253418));
#34599=DIRECTION('ref_axis',(-0.92576077253418,0.,-0.378109761890538));
#34600=DIRECTION('',(0.,1.,0.));
#34601=DIRECTION('',(-0.92576077253418,0.,-0.378109761890538));
#34602=DIRECTION('',(0.,1.,0.));
#34603=DIRECTION('center_axis',(0.,1.,0.));
#34604=DIRECTION('ref_axis',(0.,0.,1.));
#34605=DIRECTION('center_axis',(0.,1.,0.));
#34606=DIRECTION('ref_axis',(1.,0.,0.));
#34607=DIRECTION('',(0.466129625412504,0.,-0.884716436104133));
#34608=DIRECTION('center_axis',(0.884716436104133,0.,0.466129625412504));
#34609=DIRECTION('ref_axis',(0.466129625412504,0.,-0.884716436104133));
#34610=DIRECTION('',(0.,-1.,0.));
#34611=DIRECTION('center_axis',(0.671935785203096,0.,-0.740609411608777));
#34612=DIRECTION('ref_axis',(-0.740609411608777,0.,-0.671935785203096));
#34613=DIRECTION('',(0.,1.,0.));
#34614=DIRECTION('',(-0.740609411608777,0.,-0.671935785203096));
#34615=DIRECTION('',(0.,1.,0.));
#34616=DIRECTION('center_axis',(0.,1.,0.));
#34617=DIRECTION('ref_axis',(0.,0.,1.));
#34618=DIRECTION('center_axis',(0.,1.,0.));
#34619=DIRECTION('ref_axis',(1.,0.,0.));
#34620=DIRECTION('',(0.740609411608777,0.,-0.671935785203096));
#34621=DIRECTION('center_axis',(0.,1.,0.));
#34622=DIRECTION('ref_axis',(1.,0.,0.));
#34623=DIRECTION('center_axis',(0.671935785203096,0.,0.740609411608777));
#34624=DIRECTION('ref_axis',(0.740609411608777,0.,-0.671935785203096));
#34625=DIRECTION('',(0.,-1.,0.));
#34626=DIRECTION('center_axis',(0.990787227786984,0.,-0.135427727050936));
#34627=DIRECTION('ref_axis',(-0.135427727050936,0.,-0.990787227786984));
#34628=DIRECTION('',(0.,1.,0.));
#34629=DIRECTION('',(-0.135427727050936,0.,-0.990787227786984));
#34630=DIRECTION('',(0.,1.,0.));
#34631=DIRECTION('center_axis',(0.,1.,0.));
#34632=DIRECTION('ref_axis',(0.,0.,1.));
#34633=DIRECTION('center_axis',(0.,1.,0.));
#34634=DIRECTION('ref_axis',(1.,0.,0.));
#34635=DIRECTION('',(0.999251721518066,0.,-0.0386781209882463));
#34636=DIRECTION('center_axis',(0.0386781209882463,0.,0.999251721518066));
#34637=DIRECTION('ref_axis',(0.999251721518066,0.,-0.0386781209882463));
#34638=DIRECTION('',(0.,-1.,0.));
#34639=DIRECTION('center_axis',(0.846038315115844,0.,0.53312209610552));
#34640=DIRECTION('ref_axis',(0.53312209610552,0.,-0.846038315115844));
#34641=DIRECTION('',(0.,1.,0.));
#34642=DIRECTION('',(0.53312209610552,0.,-0.846038315115844));
#34643=DIRECTION('',(0.,1.,0.));
#34644=DIRECTION('center_axis',(0.,1.,0.));
#34645=DIRECTION('ref_axis',(0.,0.,1.));
#34646=DIRECTION('center_axis',(0.,1.,0.));
#34647=DIRECTION('ref_axis',(1.,0.,0.));
#34648=DIRECTION('',(0.790333045483219,0.,0.612677465896388));
#34649=DIRECTION('center_axis',(-0.612677465896388,0.,0.790333045483219));
#34650=DIRECTION('ref_axis',(0.790333045483219,0.,0.612677465896388));
#34651=DIRECTION('',(0.,-1.,0.));
#34652=DIRECTION('center_axis',(0.305418672133534,0.,0.952218165502102));
#34653=DIRECTION('ref_axis',(0.952218165502102,0.,-0.305418672133534));
#34654=DIRECTION('',(0.,1.,0.));
#34655=DIRECTION('',(0.952218165502102,0.,-0.305418672133534));
#34656=DIRECTION('',(0.,1.,0.));
#34657=DIRECTION('center_axis',(0.,1.,0.));
#34658=DIRECTION('ref_axis',(0.,0.,1.));
#34659=DIRECTION('center_axis',(0.,1.,0.));
#34660=DIRECTION('ref_axis',(1.,0.,0.));
#34661=DIRECTION('',(0.211608753893355,0.,0.977354457336591));
#34662=DIRECTION('center_axis',(-0.977354457336591,0.,0.211608753893355));
#34663=DIRECTION('ref_axis',(0.211608753893355,0.,0.977354457336591));
#34664=DIRECTION('',(0.,-1.,0.));
#34665=DIRECTION('center_axis',(-0.378109761890538,0.,0.925760772534179));
#34666=DIRECTION('ref_axis',(0.925760772534179,0.,0.378109761890538));
#34667=DIRECTION('',(0.,1.,0.));
#34668=DIRECTION('',(0.925760772534179,0.,0.378109761890538));
#34669=DIRECTION('',(0.,1.,0.));
#34670=DIRECTION('center_axis',(0.,1.,0.));
#34671=DIRECTION('ref_axis',(0.,0.,1.));
#34672=DIRECTION('center_axis',(0.,1.,0.));
#34673=DIRECTION('ref_axis',(1.,0.,0.));
#34674=DIRECTION('',(-0.4661296254125,0.,0.884716436104135));
#34675=DIRECTION('center_axis',(-0.884716436104135,0.,-0.4661296254125));
#34676=DIRECTION('ref_axis',(-0.4661296254125,0.,0.884716436104135));
#34677=DIRECTION('',(0.,-1.,0.));
#34678=DIRECTION('center_axis',(0.,-1.,0.));
#34679=DIRECTION('ref_axis',(1.,0.,0.));
#34680=DIRECTION('center_axis',(0.,-1.,0.));
#34681=DIRECTION('ref_axis',(1.,0.,0.));
#34682=DIRECTION('center_axis',(0.,-1.,0.));
#34683=DIRECTION('ref_axis',(1.,0.,0.));
#34684=DIRECTION('center_axis',(0.,-1.,0.));
#34685=DIRECTION('ref_axis',(1.,0.,0.));
#34686=DIRECTION('center_axis',(0.,-1.,0.));
#34687=DIRECTION('ref_axis',(1.,0.,0.));
#34688=DIRECTION('center_axis',(0.,-1.,0.));
#34689=DIRECTION('ref_axis',(1.,0.,0.));
#34690=DIRECTION('center_axis',(0.,-1.,0.));
#34691=DIRECTION('ref_axis',(1.,0.,0.));
#34692=DIRECTION('center_axis',(0.,-1.,0.));
#34693=DIRECTION('ref_axis',(1.,0.,0.));
#34694=DIRECTION('',(0.,1.,0.));
#34695=DIRECTION('center_axis',(0.,-1.,0.));
#34696=DIRECTION('ref_axis',(1.,0.,0.));
#34697=DIRECTION('center_axis',(0.,-1.,0.));
#34698=DIRECTION('ref_axis',(1.,0.,0.));
#34699=DIRECTION('center_axis',(0.,-1.,0.));
#34700=DIRECTION('ref_axis',(1.,0.,0.));
#34701=DIRECTION('center_axis',(0.,-1.,0.));
#34702=DIRECTION('ref_axis',(1.,0.,0.));
#34703=DIRECTION('center_axis',(0.,-1.,0.));
#34704=DIRECTION('ref_axis',(1.,0.,0.));
#34705=DIRECTION('center_axis',(0.,-1.,0.));
#34706=DIRECTION('ref_axis',(1.,0.,0.));
#34707=DIRECTION('center_axis',(0.,-1.,0.));
#34708=DIRECTION('ref_axis',(1.,0.,0.));
#34709=DIRECTION('center_axis',(0.,-1.,0.));
#34710=DIRECTION('ref_axis',(1.,0.,0.));
#34711=DIRECTION('center_axis',(0.,-1.,0.));
#34712=DIRECTION('ref_axis',(1.,0.,0.));
#34713=DIRECTION('center_axis',(0.,-1.,0.));
#34714=DIRECTION('ref_axis',(1.,0.,0.));
#34715=DIRECTION('center_axis',(0.,-1.,0.));
#34716=DIRECTION('ref_axis',(1.,0.,0.));
#34717=DIRECTION('center_axis',(0.,-1.,0.));
#34718=DIRECTION('ref_axis',(1.,0.,0.));
#34719=DIRECTION('center_axis',(0.,1.,0.));
#34720=DIRECTION('ref_axis',(0.,0.,1.));
#34721=DIRECTION('center_axis',(0.,-1.,0.));
#34722=DIRECTION('ref_axis',(1.,0.,0.));
#34723=DIRECTION('center_axis',(0.,-1.,0.));
#34724=DIRECTION('ref_axis',(1.,0.,0.));
#34725=DIRECTION('center_axis',(0.,1.,0.));
#34726=DIRECTION('ref_axis',(1.,0.,8.81908600741727E-14));
#34727=DIRECTION('center_axis',(0.,-1.,0.));
#34728=DIRECTION('ref_axis',(1.,0.,8.81908600741727E-14));
#34729=DIRECTION('center_axis',(0.,1.,0.));
#34730=DIRECTION('ref_axis',(0.,0.,1.));
#34731=DIRECTION('center_axis',(0.,-1.,0.));
#34732=DIRECTION('ref_axis',(1.,0.,0.));
#34733=DIRECTION('center_axis',(0.,-1.,0.));
#34734=DIRECTION('ref_axis',(1.,0.,0.));
#34735=DIRECTION('',(0.707106781186547,0.707106781186547,8.65956056235493E-17));
#34736=DIRECTION('center_axis',(0.,-1.,0.));
#34737=DIRECTION('ref_axis',(1.,0.,0.));
#34738=DIRECTION('center_axis',(0.,-1.,0.));
#34739=DIRECTION('ref_axis',(1.,0.,0.));
#34740=DIRECTION('center_axis',(0.,1.,0.));
#34741=DIRECTION('ref_axis',(0.,0.,1.));
#34742=DIRECTION('center_axis',(0.,-1.,0.));
#34743=DIRECTION('ref_axis',(1.,0.,0.));
#34744=DIRECTION('center_axis',(0.,-1.,0.));
#34745=DIRECTION('ref_axis',(1.,0.,0.));
#34746=DIRECTION('',(0.707106781186545,0.70710678118655,8.6595605623549E-17));
#34747=DIRECTION('center_axis',(0.,1.,0.));
#34748=DIRECTION('ref_axis',(1.,0.,0.));
#34749=DIRECTION('center_axis',(0.,-1.,0.));
#34750=DIRECTION('ref_axis',(1.,0.,0.));
#34751=DIRECTION('',(-0.447213595499958,0.894427190999916,-5.47678698264203E-17));
#34752=DIRECTION('center_axis',(0.,-1.,0.));
#34753=DIRECTION('ref_axis',(0.,0.,-1.));
#46066=CARTESIAN_POINT('',(0.,0.,0.));
#46067=CARTESIAN_POINT('Origin',(3.,-8.675,108.25));
#46068=CARTESIAN_POINT('',(2.60625649213161,-7.7837163522035,108.250229924968));
#46069=CARTESIAN_POINT('',(2.60668122837429,-7.76538364779651,108.250085965705));
#46070=CARTESIAN_POINT('',(2.6067,-8.675,108.25));
#46071=CARTESIAN_POINT('',(3.17509927743318,-7.7433,108.602463550232));
#46072=CARTESIAN_POINT('Ctrl Pts',(2.60625649213161,-7.7837163522035,108.250229924968));
#46073=CARTESIAN_POINT('Ctrl Pts',(2.60613945209692,-7.78293249916356,108.265681706531));
#46074=CARTESIAN_POINT('Ctrl Pts',(2.6069678498412,-7.78214864612363,108.281121586166));
#46075=CARTESIAN_POINT('Ctrl Pts',(2.60878318617272,-7.78136479308369,108.296444836968));
#46076=CARTESIAN_POINT('Ctrl Pts',(2.62404334187615,-7.77477553508761,108.425255784597));
#46077=CARTESIAN_POINT('Ctrl Pts',(2.70904541124582,-7.76818627709154,108.545825167833));
#46078=CARTESIAN_POINT('Ctrl Pts',(2.82537830757008,-7.76159701909547,108.603239329314));
#46079=CARTESIAN_POINT('Ctrl Pts',(2.93305584509882,-7.75549801273031,108.656381782763));
#46080=CARTESIAN_POINT('Ctrl Pts',(3.06757551455752,-7.74939900636515,108.655417116828));
#46081=CARTESIAN_POINT('Ctrl Pts',(3.17532910733319,-7.7433,108.602640901019));
#46082=CARTESIAN_POINT('',(2.82513055246694,-7.7433,108.602286199445));
#46083=CARTESIAN_POINT('Origin',(3.,-7.7433,108.25));
#46084=CARTESIAN_POINT('Ctrl Pts',(2.82513055246694,-7.7433,108.602286199445));
#46085=CARTESIAN_POINT('Ctrl Pts',(2.76678980321959,-7.74659462899803,108.573326749414));
#46086=CARTESIAN_POINT('Ctrl Pts',(2.71608793488113,-7.74988925799607,108.529614647539));
#46087=CARTESIAN_POINT('Ctrl Pts',(2.67847603852021,-7.75318388699411,108.476364995972));
#46088=CARTESIAN_POINT('Ctrl Pts',(2.64086414215929,-7.75647851599215,108.423115344405));
#46089=CARTESIAN_POINT('Ctrl Pts',(2.61634221777591,-7.75977314499018,108.360328143146));
#46090=CARTESIAN_POINT('Ctrl Pts',(2.60902703442541,-7.76306777398822,108.295710507143));
#46091=CARTESIAN_POINT('Ctrl Pts',(2.60731302843422,-7.76383973192431,108.280570077992));
#46092=CARTESIAN_POINT('Ctrl Pts',(2.6065436766476,-7.76461168986041,108.265329157535));
#46093=CARTESIAN_POINT('Ctrl Pts',(2.60668122837429,-7.76538364779651,108.250085965705));
#46094=CARTESIAN_POINT('Origin',(3.,-8.675,108.25));
#46095=CARTESIAN_POINT('',(2.6072504675668,-7.9087163522035,108.250119138638));
#46096=CARTESIAN_POINT('',(2.60725049571743,-7.8903836477965,108.250120855519));
#46097=CARTESIAN_POINT('',(2.6067,-8.675,108.25));
#46098=CARTESIAN_POINT('Ctrl Pts',(2.6072504675668,-7.9087163522035,108.250119138638));
#46099=CARTESIAN_POINT('Ctrl Pts',(2.60709204657907,-7.90580138047333,108.307959202922));
#46100=CARTESIAN_POINT('Ctrl Pts',(2.6190548870917,-7.90288640874317,108.365736924121));
#46101=CARTESIAN_POINT('Ctrl Pts',(2.64347095486817,-7.89997143701301,108.417658509612));
#46102=CARTESIAN_POINT('Ctrl Pts',(2.69866317788841,-7.89338217901694,108.535026619507));
#46103=CARTESIAN_POINT('Ctrl Pts',(2.81748896429703,-7.88679292102086,108.622471017667));
#46104=CARTESIAN_POINT('Ctrl Pts',(2.94596136011873,-7.88020366302479,108.640259746685));
#46105=CARTESIAN_POINT('Ctrl Pts',(3.07443375594042,-7.87361440502872,108.658048475703));
#46106=CARTESIAN_POINT('Ctrl Pts',(3.21255276117519,-7.86702514703264,108.60618153558));
#46107=CARTESIAN_POINT('Ctrl Pts',(3.29755898965757,-7.86043588903657,108.508227566117));
#46108=CARTESIAN_POINT('Ctrl Pts',(3.38256521813994,-7.85384663104049,108.410273596654));
#46109=CARTESIAN_POINT('Ctrl Pts',(3.41445866986993,-7.84725737304442,108.266232597851));
#46110=CARTESIAN_POINT('Ctrl Pts',(3.37875802532747,-7.84066811504835,108.141544345639));
#46111=CARTESIAN_POINT('Ctrl Pts',(3.34305738078501,-7.83407885705227,108.016856093426));
#46112=CARTESIAN_POINT('Ctrl Pts',(3.2397626399701,-7.8274895990562,107.911520587802));
#46113=CARTESIAN_POINT('Ctrl Pts',(3.1157850441026,-7.82090034106013,107.873410132177));
#46114=CARTESIAN_POINT('Ctrl Pts',(2.99180744823511,-7.81431108306405,107.835299676552));
#46115=CARTESIAN_POINT('Ctrl Pts',(2.84714699731501,-7.80772182506798,107.864414270924));
#46116=CARTESIAN_POINT('Ctrl Pts',(2.74757589287356,-7.8011325670719,107.947497824121));
#46117=CARTESIAN_POINT('Ctrl Pts',(2.65984969008155,-7.79532716211577,108.020697822025));
#46118=CARTESIAN_POINT('Ctrl Pts',(2.60712331889994,-7.78952175715963,108.135790298277));
#46119=CARTESIAN_POINT('Ctrl Pts',(2.60625649213161,-7.7837163522035,108.250229924968));
#46120=CARTESIAN_POINT('Ctrl Pts',(2.60668122837429,-7.76538364779651,108.250085965705));
#46121=CARTESIAN_POINT('Ctrl Pts',(2.60771778701373,-7.77120094785648,108.135216726595));
#46122=CARTESIAN_POINT('Ctrl Pts',(2.66025547383863,-7.77701824791646,108.020218501052));
#46123=CARTESIAN_POINT('Ctrl Pts',(2.74813923550879,-7.78283554797644,107.947123585965));
#46124=CARTESIAN_POINT('Ctrl Pts',(2.84768520586264,-7.78942480597251,107.864328947774));
#46125=CARTESIAN_POINT('Ctrl Pts',(2.99258054913982,-7.79601406396859,107.835296682375));
#46126=CARTESIAN_POINT('Ctrl Pts',(3.11653221376756,-7.80260332196466,107.873581317922));
#46127=CARTESIAN_POINT('Ctrl Pts',(3.2404838783953,-7.80919257996074,107.911865953469));
#46128=CARTESIAN_POINT('Ctrl Pts',(3.34349186437361,-7.81578183795681,108.017467489963));
#46129=CARTESIAN_POINT('Ctrl Pts',(3.37894041067353,-7.82237109595288,108.142241424483));
#46130=CARTESIAN_POINT('Ctrl Pts',(3.41438895697344,-7.82896035394896,108.267015359004));
#46131=CARTESIAN_POINT('Ctrl Pts',(3.38227806359496,-7.83554961194503,108.410961691551));
#46132=CARTESIAN_POINT('Ctrl Pts',(3.2971067528766,-7.8421388699411,108.508752957582));
#46133=CARTESIAN_POINT('Ctrl Pts',(3.21193544215825,-7.84872812793718,108.606544223614));
#46134=CARTESIAN_POINT('Ctrl Pts',(3.07370371410001,-7.85531738593325,108.65818042313));
#46135=CARTESIAN_POINT('Ctrl Pts',(2.94525789024272,-7.86190664392932,108.64016589163));
#46136=CARTESIAN_POINT('Ctrl Pts',(2.81681206638544,-7.8684959019254,108.622151360131));
#46137=CARTESIAN_POINT('Ctrl Pts',(2.69815214672911,-7.87508515992147,108.534486097616));
#46138=CARTESIAN_POINT('Ctrl Pts',(2.64317287905176,-7.88167441791754,108.417017045322));
#46139=CARTESIAN_POINT('Ctrl Pts',(2.61895026900654,-7.88457749454386,108.365262862949));
#46140=CARTESIAN_POINT('Ctrl Pts',(2.60708859829341,-7.88748057117018,108.307723519372));
#46141=CARTESIAN_POINT('Ctrl Pts',(2.60725049571743,-7.8903836477965,108.250120855519));
#46142=CARTESIAN_POINT('Origin',(3.,-8.675,108.25));
#46143=CARTESIAN_POINT('',(2.60665619608725,-8.03371635220349,108.249648010219));
#46144=CARTESIAN_POINT('',(2.60666319360669,-8.0153836477965,108.249647856379));
#46145=CARTESIAN_POINT('',(2.6067,-8.675,108.25));
#46146=CARTESIAN_POINT('Ctrl Pts',(2.60665619608725,-8.03371635220349,108.249648010219));
#46147=CARTESIAN_POINT('Ctrl Pts',(2.60755960895731,-8.02867026178311,108.349392781015));
#46148=CARTESIAN_POINT('Ctrl Pts',(2.64618731517242,-8.02362417136272,108.449760362024));
#46149=CARTESIAN_POINT('Ctrl Pts',(2.7146802163416,-8.01857808094234,108.521689468641));
#46150=CARTESIAN_POINT('Ctrl Pts',(2.80411923924929,-8.01198882294626,108.615615538418));
#46151=CARTESIAN_POINT('Ctrl Pts',(2.94448294371447,-8.00539956495019,108.661049701325));
#46152=CARTESIAN_POINT('Ctrl Pts',(3.07199651953032,-7.99881030695412,108.637348746016));
#46153=CARTESIAN_POINT('Ctrl Pts',(3.19951009534616,-7.99222104895804,108.613647790707));
#46154=CARTESIAN_POINT('Ctrl Pts',(3.31417354251268,-7.98563179096197,108.520811717183));
#46155=CARTESIAN_POINT('Ctrl Pts',(3.36388900806646,-7.97904253296589,108.401021004485));
#46156=CARTESIAN_POINT('Ctrl Pts',(3.41360447362024,-7.97245327496982,108.281230291786));
#46157=CARTESIAN_POINT('Ctrl Pts',(3.39837195756129,-7.96586401697375,108.134484939915));
#46158=CARTESIAN_POINT('Ctrl Pts',(3.32511250731495,-7.95927475897767,108.027459251154));
#46159=CARTESIAN_POINT('Ctrl Pts',(3.25185305706861,-7.9526855009816,107.920433562394));
#46160=CARTESIAN_POINT('Ctrl Pts',(3.12056667263489,-7.94609624298553,107.853127536745));
#46161=CARTESIAN_POINT('Ctrl Pts',(2.99090366781521,-7.93950698498945,107.856122064814));
#46162=CARTESIAN_POINT('Ctrl Pts',(2.86124066299552,-7.93291772699338,107.859116592884));
#46163=CARTESIAN_POINT('Ctrl Pts',(2.73320103778988,-7.9263284689973,107.932411674671));
#46164=CARTESIAN_POINT('Ctrl Pts',(2.66496055500299,-7.91973921100123,108.04270512638));
#46165=CARTESIAN_POINT('Ctrl Pts',(2.62690846039196,-7.91606492473532,108.104206696826));
#46166=CARTESIAN_POINT('Ctrl Pts',(2.60745015528707,-7.91239063846941,108.177212443997));
#46167=CARTESIAN_POINT('Ctrl Pts',(2.6072504675668,-7.9087163522035,108.250119138638));
#46168=CARTESIAN_POINT('Ctrl Pts',(2.60725049571743,-7.8903836477965,108.250120855519));
#46169=CARTESIAN_POINT('Ctrl Pts',(2.60745606496174,-7.89406982916626,108.176979876594));
#46170=CARTESIAN_POINT('Ctrl Pts',(2.62704681118361,-7.89775601053601,108.103736808611));
#46171=CARTESIAN_POINT('Ctrl Pts',(2.66533207709101,-7.90144219190577,108.042105251368));
#46172=CARTESIAN_POINT('Ctrl Pts',(2.73376915850596,-7.90803144990184,107.93193535178));
#46173=CARTESIAN_POINT('Ctrl Pts',(2.86194193703421,-7.91462070789791,107.858868394676));
#46174=CARTESIAN_POINT('Ctrl Pts',(2.99161061635252,-7.92120996589399,107.856106004432));
#46175=CARTESIAN_POINT('Ctrl Pts',(3.12127929567083,-7.92779922389006,107.853343614187));
#46176=CARTESIAN_POINT('Ctrl Pts',(3.2524438757792,-7.93438848188613,107.920885790802));
#46177=CARTESIAN_POINT('Ctrl Pts',(3.32551099973298,-7.94097773988221,108.028042927508));
#46178=CARTESIAN_POINT('Ctrl Pts',(3.39857812368676,-7.94756699787828,108.135200064214));
#46179=CARTESIAN_POINT('Ctrl Pts',(3.41354779148594,-7.95415625587435,108.28197216101));
#46180=CARTESIAN_POINT('Ctrl Pts',(3.3636176372969,-7.96074551387043,108.401673416381));
#46181=CARTESIAN_POINT('Ctrl Pts',(3.31368748310786,-7.9673347718665,108.521374671752));
#46182=CARTESIAN_POINT('Ctrl Pts',(3.1988575069306,-7.97392402986257,108.614005085698));
#46183=CARTESIAN_POINT('Ctrl Pts',(3.07130156624882,-7.98051328785865,108.637477321651));
#46184=CARTESIAN_POINT('Ctrl Pts',(2.94374562556704,-7.98710254585472,108.660949557605));
#46185=CARTESIAN_POINT('Ctrl Pts',(2.80346372038076,-7.9936918038508,108.615263615565));
#46186=CARTESIAN_POINT('Ctrl Pts',(2.71419333797958,-8.00028106184687,108.521177241524));
#46187=CARTESIAN_POINT('Ctrl Pts',(2.64599073591757,-8.00531525716341,108.449295220236));
#46188=CARTESIAN_POINT('Ctrl Pts',(2.60756338177261,-8.01034945247996,108.349162035613));
#46189=CARTESIAN_POINT('Ctrl Pts',(2.60666319360669,-8.0153836477965,108.249647856379));
#46190=CARTESIAN_POINT('Origin',(3.,-8.675,108.25));
#46191=CARTESIAN_POINT('',(2.60614453609637,-8.15871635220349,108.250198273635));
#46192=CARTESIAN_POINT('',(2.60613983983908,-8.1403836477965,108.250194790452));
#46193=CARTESIAN_POINT('',(2.6067,-8.675,108.25));
#46194=CARTESIAN_POINT('Ctrl Pts',(2.60614453609637,-8.15871635220349,108.250198273635));
#46195=CARTESIAN_POINT('Ctrl Pts',(2.60607281260588,-8.15812840108896,108.26178099959));
#46196=CARTESIAN_POINT('Ctrl Pts',(2.60653985332135,-8.15754044997442,108.273357861683));
#46197=CARTESIAN_POINT('Ctrl Pts',(2.60756455998777,-8.15695249885988,108.284885150627));
#46198=CARTESIAN_POINT('Ctrl Pts',(2.61904860420225,-8.15036324086381,108.414073239516));
#46199=CARTESIAN_POINT('Ctrl Pts',(2.70057564494174,-8.14377398286773,108.537034927215));
#46200=CARTESIAN_POINT('Ctrl Pts',(2.81510353413581,-8.13718472487166,108.597902062653));
#46201=CARTESIAN_POINT('Ctrl Pts',(2.92963142332987,-8.13059546687558,108.658769198092));
#46202=CARTESIAN_POINT('Ctrl Pts',(3.0771601609785,-8.12400620887951,108.657541781269));
#46203=CARTESIAN_POINT('Ctrl Pts',(3.19065945543724,-8.11741695088343,108.594777493984));
#46204=CARTESIAN_POINT('Ctrl Pts',(3.30415874989598,-8.11082769288736,108.532013206699));
#46205=CARTESIAN_POINT('Ctrl Pts',(3.38362860116483,-8.10423843489129,108.407712048951));
#46206=CARTESIAN_POINT('Ctrl Pts',(3.39296155340377,-8.09764917689522,108.278350765854));
#46207=CARTESIAN_POINT('Ctrl Pts',(3.4022945056427,-8.09105991889914,108.148989482756));
#46208=CARTESIAN_POINT('Ctrl Pts',(3.34149055885173,-8.08447066090307,108.01456807431));
#46209=CARTESIAN_POINT('Ctrl Pts',(3.23817623846969,-8.077881402907,107.936161462614));
#46210=CARTESIAN_POINT('Ctrl Pts',(3.13486191808765,-8.07129214491093,107.857754850918));
#46211=CARTESIAN_POINT('Ctrl Pts',(2.98903722411454,-8.06470288691485,107.835363035972));
#46212=CARTESIAN_POINT('Ctrl Pts',(2.86695820722666,-8.05811362891878,107.87915983259));
#46213=CARTESIAN_POINT('Ctrl Pts',(2.74487919033878,-8.0515243709227,107.922956629207));
#46214=CARTESIAN_POINT('Ctrl Pts',(2.64654585053613,-8.04493511292663,108.032942037388));
#46215=CARTESIAN_POINT('Ctrl Pts',(2.61663635130991,-8.03834585493055,108.159143729803));
#46216=CARTESIAN_POINT('Ctrl Pts',(2.6096317129366,-8.03680268735487,108.188699464279));
#46217=CARTESIAN_POINT('Ctrl Pts',(2.60637991933983,-8.03525951977918,108.219144613864));
#46218=CARTESIAN_POINT('Ctrl Pts',(2.60665619608725,-8.03371635220349,108.249648010219));
#46219=CARTESIAN_POINT('Ctrl Pts',(2.60666319360669,-8.0153836477965,108.249647856379));
#46220=CARTESIAN_POINT('Ctrl Pts',(2.60638512552761,-8.01693871047603,108.218907931429));
#46221=CARTESIAN_POINT('Ctrl Pts',(2.60968786881117,-8.01849377315556,108.188227071466));
#46222=CARTESIAN_POINT('Ctrl Pts',(2.61679991108365,-8.02004883583509,108.15845622412));
#46223=CARTESIAN_POINT('Ctrl Pts',(2.64693572620495,-8.02663809383116,108.0323083868));
#46224=CARTESIAN_POINT('Ctrl Pts',(2.74546621606361,-8.03322735182724,107.922499518203));
#46225=CARTESIAN_POINT('Ctrl Pts',(2.86762360807162,-8.03981660982331,107.878921763254));
#46226=CARTESIAN_POINT('Ctrl Pts',(2.98978100007963,-8.04640586781938,107.835344008305));
#46227=CARTESIAN_POINT('Ctrl Pts',(3.13556529423699,-8.05299512581546,107.857997367006));
#46228=CARTESIAN_POINT('Ctrl Pts',(3.23873881091994,-8.05958438381153,107.936589177691));
#46229=CARTESIAN_POINT('Ctrl Pts',(3.34191232760289,-8.06617364180761,108.015180988376));
#46230=CARTESIAN_POINT('Ctrl Pts',(3.40247506681144,-8.07276289980368,108.149711251046));
#46231=CARTESIAN_POINT('Ctrl Pts',(3.39291008976981,-8.07935215779975,108.279055591377));
#46232=CARTESIAN_POINT('Ctrl Pts',(3.38334511272818,-8.08594141579582,108.408399931707));
#46233=CARTESIAN_POINT('Ctrl Pts',(3.30365241943638,-8.0925306737919,108.532558349697));
#46234=CARTESIAN_POINT('Ctrl Pts',(3.19004071814446,-8.09911993178797,108.59511895181));
#46235=CARTESIAN_POINT('Ctrl Pts',(3.07642901685254,-8.10570918978405,108.657679553924));
#46236=CARTESIAN_POINT('Ctrl Pts',(2.9288983075605,-8.11229844778012,108.658642340161));
#46237=CARTESIAN_POINT('Ctrl Pts',(2.81447977625942,-8.11888770577619,108.597569866021));
#46238=CARTESIAN_POINT('Ctrl Pts',(2.70006124495835,-8.12547696377227,108.536497391881));
#46239=CARTESIAN_POINT('Ctrl Pts',(2.61875489164825,-8.13206622176834,108.413389657363));
#46240=CARTESIAN_POINT('Ctrl Pts',(2.60750259483268,-8.13865547976441,108.284181169919));
#46241=CARTESIAN_POINT('Ctrl Pts',(2.60651887963764,-8.13923153577511,108.272885311437));
#46242=CARTESIAN_POINT('Ctrl Pts',(2.60607057840048,-8.13980759178581,108.261542825702));
#46243=CARTESIAN_POINT('Ctrl Pts',(2.60613983983908,-8.1403836477965,108.250194790452));
#46244=CARTESIAN_POINT('Origin',(3.,-8.675,108.25));
#46245=CARTESIAN_POINT('',(2.60720600634845,-8.2837163522035,108.250176314706));
#46246=CARTESIAN_POINT('',(2.60720275092572,-8.2653836477965,108.250179618267));
#46247=CARTESIAN_POINT('',(2.6067,-8.675,108.25));
#46248=CARTESIAN_POINT('Ctrl Pts',(2.60720600634845,-8.2837163522035,108.250176314706));
#46249=CARTESIAN_POINT('Ctrl Pts',(2.60698604301128,-8.28099728239873,108.304114064676));
#46250=CARTESIAN_POINT('Ctrl Pts',(2.61733932470525,-8.27827821259397,108.357971006942));
#46251=CARTESIAN_POINT('Ctrl Pts',(2.63867414580283,-8.27555914278921,108.407054689178));
#46252=CARTESIAN_POINT('Ctrl Pts',(2.69037588595888,-8.26896988479313,108.526001633857));
#46253=CARTESIAN_POINT('Ctrl Pts',(2.8065680950138,-8.26238062679706,108.616917009719));
#46254=CARTESIAN_POINT('Ctrl Pts',(2.93445836245162,-8.25579136880098,108.638493039901));
#46255=CARTESIAN_POINT('Ctrl Pts',(3.06234862988944,-8.24920211080491,108.660069070083));
#46256=CARTESIAN_POINT('Ctrl Pts',(3.20193695571016,-8.24261285280884,108.612305754586));
#46257=CARTESIAN_POINT('Ctrl Pts',(3.28980080702969,-8.23602359481276,108.516904553256));
#46258=CARTESIAN_POINT('Ctrl Pts',(3.37766465834923,-8.22943433681669,108.421503351926));
#46259=CARTESIAN_POINT('Ctrl Pts',(3.41380403516758,-8.22284507882062,108.278464264762));
#46260=CARTESIAN_POINT('Ctrl Pts',(3.38179886222579,-8.21625582082454,108.152777692334));
#46261=CARTESIAN_POINT('Ctrl Pts',(3.34979368928399,-8.20966656282847,108.027091119906));
#46262=CARTESIAN_POINT('Ctrl Pts',(3.24964396658204,-8.2030773048324,107.918757062214));
#46263=CARTESIAN_POINT('Ctrl Pts',(3.12685313465012,-8.19648804683632,107.876997546212));
#46264=CARTESIAN_POINT('Ctrl Pts',(3.00406230271819,-8.18989878884025,107.835238030209));
#46265=CARTESIAN_POINT('Ctrl Pts',(2.85863036155628,-8.18330953084418,107.860053055896));
#46266=CARTESIAN_POINT('Ctrl Pts',(2.75663491482005,-8.1767202728481,107.940167813778));
#46267=CARTESIAN_POINT('Ctrl Pts',(2.6637403921366,-8.17071896596657,108.013134033659));
#46268=CARTESIAN_POINT('Ctrl Pts',(2.60687662872517,-8.16471765908503,108.131971619654));
#46269=CARTESIAN_POINT('Ctrl Pts',(2.60614453609637,-8.15871635220349,108.250198273635));
#46270=CARTESIAN_POINT('Ctrl Pts',(2.60613983983908,-8.1403836477965,108.250194790452));
#46271=CARTESIAN_POINT('Ctrl Pts',(2.60686283033371,-8.14639684978188,108.131737510561));
#46272=CARTESIAN_POINT('Ctrl Pts',(2.66398140619207,-8.15241005176726,108.012675534682));
#46273=CARTESIAN_POINT('Ctrl Pts',(2.75719105092667,-8.15842325375264,107.939731761829));
#46274=CARTESIAN_POINT('Ctrl Pts',(2.85933004415725,-8.16501251174871,107.859800081552));
#46275=CARTESIAN_POINT('Ctrl Pts',(3.00480627093945,-8.17160176974478,107.835245961367));
#46276=CARTESIAN_POINT('Ctrl Pts',(3.1275220064063,-8.17819102774086,107.87722566715));
#46277=CARTESIAN_POINT('Ctrl Pts',(3.25023774187315,-8.18478028573693,107.919205372932));
#46278=CARTESIAN_POINT('Ctrl Pts',(3.35019298602466,-8.191369543733,108.027718904682));
#46279=CARTESIAN_POINT('Ctrl Pts',(3.38197266039813,-8.19795880172908,108.153462690723));
#46280=CARTESIAN_POINT('Ctrl Pts',(3.4137523347716,-8.20454805972515,108.279206476764));
#46281=CARTESIAN_POINT('Ctrl Pts',(3.37735643936704,-8.21113731772122,108.422180517097));
#46282=CARTESIAN_POINT('Ctrl Pts',(3.28932159975375,-8.2177265757173,108.517423965421));
#46283=CARTESIAN_POINT('Ctrl Pts',(3.20128676014047,-8.22431583371337,108.612667413746));
#46284=CARTESIAN_POINT('Ctrl Pts',(3.06161297631846,-8.23090509170945,108.660180270062));
#46285=CARTESIAN_POINT('Ctrl Pts',(2.93376160935407,-8.23749434970552,108.638374871702));
#46286=CARTESIAN_POINT('Ctrl Pts',(2.80591024238967,-8.24408360770159,108.616569473341));
#46287=CARTESIAN_POINT('Ctrl Pts',(2.6898812922829,-8.25067286569767,108.525445820303));
#46288=CARTESIAN_POINT('Ctrl Pts',(2.63839299217811,-8.25726212369374,108.406406321039));
#46289=CARTESIAN_POINT('Ctrl Pts',(2.61723919557154,-8.25996929839466,108.35749933925));
#46290=CARTESIAN_POINT('Ctrl Pts',(2.60697953705813,-8.26267647309558,108.303880302597));
#46291=CARTESIAN_POINT('Ctrl Pts',(2.60720275092572,-8.2653836477965,108.250179618267));
#46292=CARTESIAN_POINT('Origin',(3.,-8.675,108.25));
#46293=CARTESIAN_POINT('',(2.60677025899564,-8.40871635220349,108.249651168915));
#46294=CARTESIAN_POINT('',(2.60677702480763,-8.3903836477965,108.249651743722));
#46295=CARTESIAN_POINT('',(2.6067,-8.675,108.25));
#46296=CARTESIAN_POINT('Ctrl Pts',(2.60677025899564,-8.40871635220349,108.249651168915));
#46297=CARTESIAN_POINT('Ctrl Pts',(2.60760908356072,-8.40386616370851,108.345594615925));
#46298=CARTESIAN_POINT('Ctrl Pts',(2.64301678385761,-8.39901597521352,108.442092426262));
#46299=CARTESIAN_POINT('Ctrl Pts',(2.70677980611443,-8.39416578671853,108.513143432754));
#46300=CARTESIAN_POINT('Ctrl Pts',(2.79340551245423,-8.38757652872246,108.609670281791));
#46301=CARTESIAN_POINT('Ctrl Pts',(2.93236599521414,-8.38098727072638,108.659230540508));
#46302=CARTESIAN_POINT('Ctrl Pts',(3.06052398459853,-8.37439801273031,108.639306300479));
#46303=CARTESIAN_POINT('Ctrl Pts',(3.18868197398291,-8.36780875473423,108.619382060449));
#46304=CARTESIAN_POINT('Ctrl Pts',(3.30603746999177,-8.36121949673816,108.529973321673));
#46305=CARTESIAN_POINT('Ctrl Pts',(3.35926951787344,-8.35463023874209,108.411703314224));
#46306=CARTESIAN_POINT('Ctrl Pts',(3.41250156575511,-8.34804098074602,108.293433306774));
#46307=CARTESIAN_POINT('Ctrl Pts',(3.40161016550959,-8.34145172274994,108.146302030651));
#46308=CARTESIAN_POINT('Ctrl Pts',(3.33154386986275,-8.33486246475387,108.037159189392));
#46309=CARTESIAN_POINT('Ctrl Pts',(3.26147757421591,-8.3282732067578,107.928016348133));
#46310=CARTESIAN_POINT('Ctrl Pts',(3.13223638316774,-8.32168394876172,107.856861941737));
#46311=CARTESIAN_POINT('Ctrl Pts',(3.0025415661458,-8.31509469076565,107.8560252689));
#46312=CARTESIAN_POINT('Ctrl Pts',(2.87284674912387,-8.30850543276957,107.855188596062));
#46313=CARTESIAN_POINT('Ctrl Pts',(2.74269830612817,-8.3019161747735,107.924669656782));
#46314=CARTESIAN_POINT('Ctrl Pts',(2.6712297202589,-8.29532691677743,108.032899443891));
#46315=CARTESIAN_POINT('Ctrl Pts',(2.62925278184706,-8.29145672858612,108.096468004155));
#46316=CARTESIAN_POINT('Ctrl Pts',(2.60751909117935,-8.28758654039481,108.173404014622));
#46317=CARTESIAN_POINT('Ctrl Pts',(2.60720600634845,-8.2837163522035,108.250176314706));
#46318=CARTESIAN_POINT('Ctrl Pts',(2.60720275092572,-8.2653836477965,108.250179618267));
#46319=CARTESIAN_POINT('Ctrl Pts',(2.60752283918096,-8.26926573109165,108.173172940604));
#46320=CARTESIAN_POINT('Ctrl Pts',(2.62939938691649,-8.27314781438681,108.095998366703));
#46321=CARTESIAN_POINT('Ctrl Pts',(2.67161965273307,-8.27702989768196,108.032310053299));
#46322=CARTESIAN_POINT('Ctrl Pts',(2.74328226349561,-8.28361915567803,107.924208630312));
#46323=CARTESIAN_POINT('Ctrl Pts',(2.87355513512348,-8.29020841367411,107.85496112983));
#46324=CARTESIAN_POINT('Ctrl Pts',(3.00324824985443,-8.29679767167018,107.856030439959));
#46325=CARTESIAN_POINT('Ctrl Pts',(3.13294136458537,-8.30338692966625,107.857099750088));
#46326=CARTESIAN_POINT('Ctrl Pts',(3.26205472241938,-8.30997618766233,107.928485870829));
#46327=CARTESIAN_POINT('Ctrl Pts',(3.3319251354776,-8.3165654456584,108.037754223118));
#46328=CARTESIAN_POINT('Ctrl Pts',(3.40179554853582,-8.32315470365447,108.147022575406));
#46329=CARTESIAN_POINT('Ctrl Pts',(3.41242301681823,-8.32974396165055,108.294173159243));
#46330=CARTESIAN_POINT('Ctrl Pts',(3.35897890617778,-8.33633321964662,108.41234749855));
#46331=CARTESIAN_POINT('Ctrl Pts',(3.30553479553734,-8.3429224776427,108.530521837857));
#46332=CARTESIAN_POINT('Ctrl Pts',(3.18801910597402,-8.34951173563877,108.619719932635));
#46333=CARTESIAN_POINT('Ctrl Pts',(3.05982557684307,-8.35610099363485,108.639414259782));
#46334=CARTESIAN_POINT('Ctrl Pts',(2.93163204771212,-8.36269025163092,108.659108586929));
#46335=CARTESIAN_POINT('Ctrl Pts',(2.79276067901352,-8.36927950962699,108.609299146445));
#46336=CARTESIAN_POINT('Ctrl Pts',(2.70630825120084,-8.37586876762306,108.512617063523));
#46337=CARTESIAN_POINT('Ctrl Pts',(2.64282884116956,-8.38070706101421,108.441626326308));
#46338=CARTESIAN_POINT('Ctrl Pts',(2.6076112180575,-8.38554535440536,108.345364101143));
#46339=CARTESIAN_POINT('Ctrl Pts',(2.60677702480763,-8.3903836477965,108.249651743722));
#46340=CARTESIAN_POINT('Origin',(3.,-8.675,108.25));
#46341=CARTESIAN_POINT('',(2.60607704946663,-8.53371635220349,108.250137347263));
#46342=CARTESIAN_POINT('',(2.60607363302738,-8.5153836477965,108.250133427664));
#46343=CARTESIAN_POINT('',(2.6067,-8.675,108.25));
#46344=CARTESIAN_POINT('Ctrl Pts',(2.60607704946663,-8.53371635220349,108.250137347263));
#46345=CARTESIAN_POINT('Ctrl Pts',(2.6060419851575,-8.53332430301436,108.257857266924));
#46346=CARTESIAN_POINT('Ctrl Pts',(2.60624943432723,-8.53293225382521,108.265575266175));
#46347=CARTESIAN_POINT('Ctrl Pts',(2.60670538132437,-8.53254020463607,108.273278557188));
#46348=CARTESIAN_POINT('Ctrl Pts',(2.61436858400385,-8.52595094664,108.402749484073));
#46349=CARTESIAN_POINT('Ctrl Pts',(2.69222813183566,-8.51936168864393,108.528065587685));
#46350=CARTESIAN_POINT('Ctrl Pts',(2.80490821739606,-8.51277243064786,108.592288978298));
#46351=CARTESIAN_POINT('Ctrl Pts',(2.91758830295647,-8.50618317265178,108.656512368912));
#46352=CARTESIAN_POINT('Ctrl Pts',(3.06508892624547,-8.49959391465571,108.659643046527));
#46353=CARTESIAN_POINT('Ctrl Pts',(3.18039256931364,-8.49300465665963,108.600258574828));
#46354=CARTESIAN_POINT('Ctrl Pts',(3.29569621238182,-8.48641539866356,108.540874103128));
#46355=CARTESIAN_POINT('Ctrl Pts',(3.37880287522917,-8.47982614066749,108.418974482114));
#46356=CARTESIAN_POINT('Ctrl Pts',(3.39195270203343,-8.47323688267141,108.289945308519));
#46357=CARTESIAN_POINT('Ctrl Pts',(3.40510252883768,-8.46664762467534,108.160916134923));
#46358=CARTESIAN_POINT('Ctrl Pts',(3.34829551959883,-8.46005836667926,108.024757408745));
#46359=CARTESIAN_POINT('Ctrl Pts',(3.24734217380106,-8.45346910868319,107.943333410096));
#46360=CARTESIAN_POINT('Ctrl Pts',(3.14638882800329,-8.44687985068712,107.861909411447));
#46361=CARTESIAN_POINT('Ctrl Pts',(3.0012891456466,-8.44029059269105,107.835220140326));
#46362=CARTESIAN_POINT('Ctrl Pts',(2.87796976724249,-8.43370133469497,107.875391977399));
#46363=CARTESIAN_POINT('Ctrl Pts',(2.75465038883837,-8.4271120766989,107.915563814472));
#46364=CARTESIAN_POINT('Ctrl Pts',(2.65311131438682,-8.42052281870282,108.022596759739));
#46365=CARTESIAN_POINT('Ctrl Pts',(2.61948724212089,-8.41393356070675,108.14785995205));
#46366=CARTESIAN_POINT('Ctrl Pts',(2.61061301096849,-8.41219449120566,108.180920032182));
#46367=CARTESIAN_POINT('Ctrl Pts',(2.60646949249566,-8.41045542170458,108.215249965189));
#46368=CARTESIAN_POINT('Ctrl Pts',(2.60677025899564,-8.40871635220349,108.249651168915));
#46369=CARTESIAN_POINT('Ctrl Pts',(2.60677702480763,-8.3903836477965,108.249651743722));
#46370=CARTESIAN_POINT('Ctrl Pts',(2.60647513264523,-8.39213461240143,108.215013714039));
#46371=CARTESIAN_POINT('Ctrl Pts',(2.61067642280362,-8.39388557700636,108.180447700287));
#46372=CARTESIAN_POINT('Ctrl Pts',(2.61967104589793,-8.39563654161128,108.147177570357));
#46373=CARTESIAN_POINT('Ctrl Pts',(2.65351975533446,-8.40222579960736,108.021974885472));
#46374=CARTESIAN_POINT('Ctrl Pts',(2.75525066113429,-8.40881505760343,107.915124241063));
#46375=CARTESIAN_POINT('Ctrl Pts',(2.87864190569828,-8.4154043155995,107.87517366913));
#46376=CARTESIAN_POINT('Ctrl Pts',(3.00203315026227,-8.42199357359558,107.835223097197));
#46377=CARTESIAN_POINT('Ctrl Pts',(3.14708473359041,-8.42858283159165,107.86217259774));
#46378=CARTESIAN_POINT('Ctrl Pts',(3.24789186916368,-8.43517208958773,107.94377755378));
#46379=CARTESIAN_POINT('Ctrl Pts',(3.34869900473694,-8.4417613475838,108.025382509821));
#46380=CARTESIAN_POINT('Ctrl Pts',(3.40526169255533,-8.44835060557987,108.161642921358));
#46381=CARTESIAN_POINT('Ctrl Pts',(3.39188044158204,-8.45493986357595,108.290648307118));
#46382=CARTESIAN_POINT('Ctrl Pts',(3.37849919060876,-8.46152912157202,108.419653692879));
#46383=CARTESIAN_POINT('Ctrl Pts',(3.29517400084382,-8.4681183795681,108.541404052863));
#46384=CARTESIAN_POINT('Ctrl Pts',(3.17976401671787,-8.47470763756417,108.600581607703));
#46385=CARTESIAN_POINT('Ctrl Pts',(3.06435403259193,-8.48129689556024,108.659759162543));
#46386=CARTESIAN_POINT('Ctrl Pts',(2.91685925410498,-8.48788615355631,108.65636391224));
#46387=CARTESIAN_POINT('Ctrl Pts',(2.80429454359648,-8.49447541155238,108.591938502804));
#46388=CARTESIAN_POINT('Ctrl Pts',(2.69172983308797,-8.50106466954846,108.527513093369));
#46389=CARTESIAN_POINT('Ctrl Pts',(2.6140951905579,-8.50765392754453,108.4020575248));
#46390=CARTESIAN_POINT('Ctrl Pts',(2.60666423677642,-8.51424318554061,108.272573053304));
#46391=CARTESIAN_POINT('Ctrl Pts',(2.60623552273314,-8.51462333962591,108.265102705224));
#46392=CARTESIAN_POINT('Ctrl Pts',(2.60604048045085,-8.51500349371121,108.25761894701));
#46393=CARTESIAN_POINT('Ctrl Pts',(2.60607363302738,-8.5153836477965,108.250133427664));
#46394=CARTESIAN_POINT('Origin',(3.,-8.675,108.25));
#46395=CARTESIAN_POINT('',(2.60714512931118,-8.6587163522035,108.250227864382));
#46396=CARTESIAN_POINT('',(2.60714090487912,-8.6403836477965,108.250230780684));
#46397=CARTESIAN_POINT('',(2.6067,-8.675,108.25));
#46398=CARTESIAN_POINT('Ctrl Pts',(2.60714512931118,-8.6587163522035,108.250227864382));
#46399=CARTESIAN_POINT('Ctrl Pts',(2.60687884329338,-8.65619318432413,108.300260095951));
#46400=CARTESIAN_POINT('Ctrl Pts',(2.61574913749029,-8.65367001644477,108.350201453516));
#46401=CARTESIAN_POINT('Ctrl Pts',(2.63419286977669,-8.6511468485654,108.39631367599));
#46402=CARTESIAN_POINT('Ctrl Pts',(2.68235871376967,-8.64455759056933,108.516735837805));
#46403=CARTESIAN_POINT('Ctrl Pts',(2.79581485758624,-8.63796833257325,108.611043517467));
#46404=CARTESIAN_POINT('Ctrl Pts',(2.92301203326297,-8.63137907457718,108.63638763086));
#46405=CARTESIAN_POINT('Ctrl Pts',(3.05020920893969,-8.6247898165811,108.661731744253));
#46406=CARTESIAN_POINT('Ctrl Pts',(3.19114741647657,-8.61820055858503,108.618112291376));
#46407=CARTESIAN_POINT('Ctrl Pts',(3.28179079864977,-8.61161130058896,108.525347950964));
#46408=CARTESIAN_POINT('Ctrl Pts',(3.37243418082296,-8.60502204259289,108.432583610553));
#46409=CARTESIAN_POINT('Ctrl Pts',(3.41278273763247,-8.59843278459681,108.290674382606));
#46410=CARTESIAN_POINT('Ctrl Pts',(3.38450393549355,-8.59184352660074,108.164097311486));
#46411=CARTESIAN_POINT('Ctrl Pts',(3.35622513335464,-8.58525426860466,108.037520240366));
#46412=CARTESIAN_POINT('Ctrl Pts',(3.25931897226731,-8.57866501060859,107.926275326072));
#46413=CARTESIAN_POINT('Ctrl Pts',(3.13781516712542,-8.57207575261252,107.880907155293));
#46414=CARTESIAN_POINT('Ctrl Pts',(3.01631136198352,-8.56548649461644,107.835538984514));
#46415=CARTESIAN_POINT('Ctrl Pts',(2.87020991278705,-8.55889723662037,107.85604755725));
#46416=CARTESIAN_POINT('Ctrl Pts',(2.76589261695239,-8.5523079786243,107.933114718697));
#46417=CARTESIAN_POINT('Ctrl Pts',(2.66778201559982,-8.54611076981736,108.005596520431));
#46418=CARTESIAN_POINT('Ctrl Pts',(2.60663131880675,-8.53991356101043,108.128106858646));
#46419=CARTESIAN_POINT('Ctrl Pts',(2.60607704946663,-8.53371635220349,108.250137347263));
#46420=CARTESIAN_POINT('Ctrl Pts',(2.60607363302738,-8.5153836477965,108.250133427664));
#46421=CARTESIAN_POINT('Ctrl Pts',(2.60661511817905,-8.52159275170728,108.127871510083));
#46422=CARTESIAN_POINT('Ctrl Pts',(2.66803236211992,-8.52780185561805,108.005139773665));
#46423=CARTESIAN_POINT('Ctrl Pts',(2.76646139004698,-8.53401095952883,107.932695283635));
#46424=CARTESIAN_POINT('Ctrl Pts',(2.87091676213192,-8.54060021752491,107.855815359888));
#46425=CARTESIAN_POINT('Ctrl Pts',(3.01705477133471,-8.54718947552098,107.835568886818));
#46426=CARTESIAN_POINT('Ctrl Pts',(3.13847700904895,-8.55377873351705,107.881154933162));
#46427=CARTESIAN_POINT('Ctrl Pts',(3.25989924676319,-8.56036799151313,107.926740979506));
#46428=CARTESIAN_POINT('Ctrl Pts',(3.35660571298888,-8.5669572495092,108.038159545264));
#46429=CARTESIAN_POINT('Ctrl Pts',(3.38465742501809,-8.57354650750527,108.164787144488));
#46430=CARTESIAN_POINT('Ctrl Pts',(3.4127091370473,-8.58013576550134,108.291414743711));
#46431=CARTESIAN_POINT('Ctrl Pts',(3.37210609488002,-8.58672502349742,108.433251376399));
#46432=CARTESIAN_POINT('Ctrl Pts',(3.28129645857532,-8.59331428149349,108.525852982146));
#46433=CARTESIAN_POINT('Ctrl Pts',(3.19048682227062,-8.59990353948957,108.618454587894));
#46434=CARTESIAN_POINT('Ctrl Pts',(3.0494705918285,-8.60649279748564,108.661821166701));
#46435=CARTESIAN_POINT('Ctrl Pts',(2.92231907450233,-8.61308205548171,108.636248934212));
#46436=CARTESIAN_POINT('Ctrl Pts',(2.79516755717617,-8.61967131347779,108.610676701723));
#46437=CARTESIAN_POINT('Ctrl Pts',(2.68188075296595,-8.62626057147386,108.516165657938));
#46438=CARTESIAN_POINT('Ctrl Pts',(2.63393098968494,-8.63284982946993,108.395657286303));
#46439=CARTESIAN_POINT('Ctrl Pts',(2.61565655951509,-8.63536110224546,108.349729597162));
#46440=CARTESIAN_POINT('Ctrl Pts',(2.60687230419797,-8.63787237502098,108.300025808225));
#46441=CARTESIAN_POINT('Ctrl Pts',(2.60714090487912,-8.6403836477965,108.250230780684));
#46442=CARTESIAN_POINT('Origin',(3.,-8.675,108.25));
#46443=CARTESIAN_POINT('',(2.60687901882508,-8.78371635220349,108.249666035988));
#46444=CARTESIAN_POINT('',(2.60688536129284,-8.7653836477965,108.249667300834));
#46445=CARTESIAN_POINT('',(2.6067,-8.675,108.25));
#46446=CARTESIAN_POINT('Ctrl Pts',(2.60687901882508,-8.78371635220349,108.249666035988));
#46447=CARTESIAN_POINT('Ctrl Pts',(2.6076329537605,-8.7790620656339,108.341799007699));
#46448=CARTESIAN_POINT('Ctrl Pts',(2.63998823948557,-8.77440777906431,108.434409003843));
#46449=CARTESIAN_POINT('Ctrl Pts',(2.69913526959871,-8.76975349249472,108.504367769783));
#46450=CARTESIAN_POINT('Ctrl Pts',(2.78287206476371,-8.76316423449865,108.603411167944));
#46451=CARTESIAN_POINT('Ctrl Pts',(2.92030805502711,-8.75657497650258,108.65705428114));
#46452=CARTESIAN_POINT('Ctrl Pts',(3.0489986300612,-8.7499857185065,108.640924139132));
#46453=CARTESIAN_POINT('Ctrl Pts',(3.1776892050953,-8.74339646051043,108.624793997124));
#46454=CARTESIAN_POINT('Ctrl Pts',(3.2976343649001,-8.73680720251436,108.538890599913));
#46455=CARTESIAN_POINT('Ctrl Pts',(3.35433653027273,-8.73021794451828,108.422244511141));
#46456=CARTESIAN_POINT('Ctrl Pts',(3.41103869564537,-8.72362868652221,108.305598422369));
#46457=CARTESIAN_POINT('Ctrl Pts',(3.40449786658584,-8.71703942852613,108.158209642035));
#46458=CARTESIAN_POINT('Ctrl Pts',(3.33768589581671,-8.71045017053006,108.047044871781));
#46459=CARTESIAN_POINT('Ctrl Pts',(3.27087392504758,-8.70386091253399,107.935880101526));
#46460=CARTESIAN_POINT('Ctrl Pts',(3.14379081256885,-8.69727165453792,107.860939341351));
#46461=CARTESIAN_POINT('Ctrl Pts',(3.01417729588862,-8.69068239654184,107.85627223544));
#46462=CARTESIAN_POINT('Ctrl Pts',(2.8845637792084,-8.68409313854577,107.85160512953));
#46463=CARTESIAN_POINT('Ctrl Pts',(2.75241985832666,-8.6775038805497,107.917211677884));
#46464=CARTESIAN_POINT('Ctrl Pts',(2.67778566997049,-8.67091462255362,108.023283274045));
#46465=CARTESIAN_POINT('Ctrl Pts',(2.63173050930985,-8.66684853243691,108.088737786385));
#46466=CARTESIAN_POINT('Ctrl Pts',(2.6075742497649,-8.66278244232021,108.169600822494));
#46467=CARTESIAN_POINT('Ctrl Pts',(2.60714512931118,-8.6587163522035,108.250227864382));
#46468=CARTESIAN_POINT('Ctrl Pts',(2.60714090487912,-8.6403836477965,108.250230780684));
#46469=CARTESIAN_POINT('Ctrl Pts',(2.60757707796976,-8.64446163301706,108.169370036145));
#46470=CARTESIAN_POINT('Ctrl Pts',(2.63188526888634,-8.64853961823761,108.088268699072));
#46471=CARTESIAN_POINT('Ctrl Pts',(2.67819284115219,-8.65261760345816,108.022705658054));
#46472=CARTESIAN_POINT('Ctrl Pts',(2.75301717825226,-8.65920686145423,107.916768100926));
#46473=CARTESIAN_POINT('Ctrl Pts',(2.88527857480418,-8.6657961194503,107.851398686154));
#46474=CARTESIAN_POINT('Ctrl Pts',(3.01488351852452,-8.67238537744638,107.856298277572));
#46475=CARTESIAN_POINT('Ctrl Pts',(3.14448846224486,-8.67897463544245,107.861197868991));
#46476=CARTESIAN_POINT('Ctrl Pts',(3.27143695313361,-8.68556389343853,107.936366466601));
#46477=CARTESIAN_POINT('Ctrl Pts',(3.33804941955861,-8.6921531514346,108.047650907335));
#46478=CARTESIAN_POINT('Ctrl Pts',(3.4046618859836,-8.69874240943067,108.15893534807));
#46479=CARTESIAN_POINT('Ctrl Pts',(3.41093832794482,-8.70533166742674,108.306335631929));
#46480=CARTESIAN_POINT('Ctrl Pts',(3.3540270180908,-8.71192092542282,108.422879830599));
#46481=CARTESIAN_POINT('Ctrl Pts',(3.29711570823677,-8.71851018341889,108.539424029268));
#46482=CARTESIAN_POINT('Ctrl Pts',(3.17701664656749,-8.72509944141497,108.625112142748));
#46483=CARTESIAN_POINT('Ctrl Pts',(3.04829733823417,-8.73168869941104,108.641011422449));
#46484=CARTESIAN_POINT('Ctrl Pts',(2.91957802990085,-8.73827795740711,108.65691070215));
#46485=CARTESIAN_POINT('Ctrl Pts',(2.78223847490348,-8.74486721540318,108.603021148073));
#46486=CARTESIAN_POINT('Ctrl Pts',(2.69867946780799,-8.75145647339926,108.503827701888));
#46487=CARTESIAN_POINT('Ctrl Pts',(2.63980886027409,-8.75609886486501,108.43394201699));
#46488=CARTESIAN_POINT('Ctrl Pts',(2.6076336087024,-8.76074125633075,108.341568581902));
#46489=CARTESIAN_POINT('Ctrl Pts',(2.60688536129284,-8.7653836477965,108.249667300834));
#46490=CARTESIAN_POINT('Origin',(3.,-8.675,108.25));
#46491=CARTESIAN_POINT('',(2.60603291882732,-8.9087163522035,108.250070364255));
#46492=CARTESIAN_POINT('',(2.60603107819738,-8.8903836477965,108.250066160239));
#46493=CARTESIAN_POINT('',(2.6067,-8.675,108.25));
#46494=CARTESIAN_POINT('Ctrl Pts',(2.60603291882732,-8.9087163522035,108.250070364255));
#46495=CARTESIAN_POINT('Ctrl Pts',(2.60602332688793,-8.90852020493976,108.253931583289));
#46496=CARTESIAN_POINT('Ctrl Pts',(2.60607522236371,-8.90832405767601,108.257792538181));
#46497=CARTESIAN_POINT('Ctrl Pts',(2.60618940167944,-8.90812791041227,108.261651650285));
#46498=CARTESIAN_POINT('Ctrl Pts',(2.61002507572765,-8.9015386524162,108.391292435489));
#46499=CARTESIAN_POINT('Ctrl Pts',(2.6841491884467,-8.89494939442012,108.518853600922));
#46500=CARTESIAN_POINT('Ctrl Pts',(2.79488314279838,-8.88836013642405,108.58637720374));
#46501=CARTESIAN_POINT('Ctrl Pts',(2.90561709715007,-8.88177087842798,108.653900806557));
#46502=CARTESIAN_POINT('Ctrl Pts',(3.0529608931344,-8.8751816204319,108.661386846759));
#46503=CARTESIAN_POINT('Ctrl Pts',(3.16996826793614,-8.86859236243583,108.605434011033));
#46504=CARTESIAN_POINT('Ctrl Pts',(3.28697564273788,-8.86200310443976,108.549481175306));
#46505=CARTESIAN_POINT('Ctrl Pts',(3.37364659635704,-8.85541384644368,108.430089463652));
#46506=CARTESIAN_POINT('Ctrl Pts',(3.39060182272462,-8.84882458844761,108.301504993818));
#46507=CARTESIAN_POINT('Ctrl Pts',(3.40755704909219,-8.84223533045154,108.172920523983));
#46508=CARTESIAN_POINT('Ctrl Pts',(3.35479654820819,-8.83564607245546,108.035143295968));
#46509=CARTESIAN_POINT('Ctrl Pts',(3.25629227175775,-8.82905681445939,107.950772962884));
#46510=CARTESIAN_POINT('Ctrl Pts',(3.15778799530732,-8.82246755646331,107.8664026298));
#46511=CARTESIAN_POINT('Ctrl Pts',(3.01353994329047,-8.81587829846724,107.835439191646));
#46512=CARTESIAN_POINT('Ctrl Pts',(2.88908781445318,-8.80928904047117,107.871951014548));
#46513=CARTESIAN_POINT('Ctrl Pts',(2.7646356856159,-8.80269978247509,107.908462837451));
#46514=CARTESIAN_POINT('Ctrl Pts',(2.65997947995819,-8.79611052447902,108.01244992141));
#46515=CARTESIAN_POINT('Ctrl Pts',(2.62267017716264,-8.78952126648294,108.136665304953));
#46516=CARTESIAN_POINT('Ctrl Pts',(2.61171409760188,-8.78758629505646,108.173141827503));
#46517=CARTESIAN_POINT('Ctrl Pts',(2.60656557818587,-8.78565132362998,108.211362707425));
#46518=CARTESIAN_POINT('Ctrl Pts',(2.60687901882508,-8.78371635220349,108.249666035988));
#46519=CARTESIAN_POINT('Ctrl Pts',(2.60688536129284,-8.7653836477965,108.249667300834));
#46520=CARTESIAN_POINT('Ctrl Pts',(2.60657157090079,-8.76733051432683,108.21112692148));
#46521=CARTESIAN_POINT('Ctrl Pts',(2.61178481051869,-8.76927738085715,108.172669579293));
#46522=CARTESIAN_POINT('Ctrl Pts',(2.62287405626398,-8.77122424738748,108.135988650006));
#46523=CARTESIAN_POINT('Ctrl Pts',(2.66040611100908,-8.77781350538355,108.011840382602));
#46524=CARTESIAN_POINT('Ctrl Pts',(2.7652486796929,-8.78440276337963,107.908041186087));
#46525=CARTESIAN_POINT('Ctrl Pts',(2.88976610782154,-8.7909920213757,107.871752654495));
#46526=CARTESIAN_POINT('Ctrl Pts',(3.01428353595017,-8.79758127937177,107.835464122904));
#46527=CARTESIAN_POINT('Ctrl Pts',(3.15847582352362,-8.80417053736785,107.866686256237));
#46528=CARTESIAN_POINT('Ctrl Pts',(3.25682860860126,-8.81075979536392,107.951233149145));
#46529=CARTESIAN_POINT('Ctrl Pts',(3.35518139367891,-8.81734905335999,108.035780042052));
#46530=CARTESIAN_POINT('Ctrl Pts',(3.40769467626076,-8.82393831135607,108.173651694534));
#46531=CARTESIAN_POINT('Ctrl Pts',(3.39050882931922,-8.83052756935214,108.302205551332));
#46532=CARTESIAN_POINT('Ctrl Pts',(3.37332298237768,-8.83711682734822,108.43075940813));
#46533=CARTESIAN_POINT('Ctrl Pts',(3.28643800591276,-8.84370608534429,108.549995469245));
#46534=CARTESIAN_POINT('Ctrl Pts',(3.16933044815818,-8.85029534334036,108.605738337395));
#46535=CARTESIAN_POINT('Ctrl Pts',(3.0522228904036,-8.85688460133643,108.661481205545));
#46536=CARTESIAN_POINT('Ctrl Pts',(2.90489275135936,-8.86347385933251,108.65373088073));
#46537=CARTESIAN_POINT('Ctrl Pts',(2.7942800887535,-8.87006311732858,108.586008755069));
#46538=CARTESIAN_POINT('Ctrl Pts',(2.68366742614764,-8.87665237532465,108.518286629408));
#46539=CARTESIAN_POINT('Ctrl Pts',(2.60977223998017,-8.88324163332073,108.3905927029));
#46540=CARTESIAN_POINT('Ctrl Pts',(2.6061691135642,-8.8898308913168,108.260945238934));
#46541=CARTESIAN_POINT('Ctrl Pts',(2.60606836112365,-8.8900151434767,108.25731997107));
#46542=CARTESIAN_POINT('Ctrl Pts',(2.60602257016326,-8.8901993956366,108.253693175732));
#46543=CARTESIAN_POINT('Ctrl Pts',(2.60603107819738,-8.8903836477965,108.250066160239));
#46544=CARTESIAN_POINT('Origin',(3.,-8.675,108.25));
#46545=CARTESIAN_POINT('',(2.60706905675086,-9.03371635220349,108.250272277881));
#46546=CARTESIAN_POINT('',(2.60706396640167,-9.0153836477965,108.250274710706));
#46547=CARTESIAN_POINT('',(2.6067,-8.675,108.25));
#46548=CARTESIAN_POINT('Ctrl Pts',(2.60706905675086,-9.03371635220349,108.250272277881));
#46549=CARTESIAN_POINT('Ctrl Pts',(2.60677194109989,-9.03138908624953,108.296397492467));
#46550=CARTESIAN_POINT('Ctrl Pts',(2.61428275998129,-9.02906182029556,108.342429055414));
#46551=CARTESIAN_POINT('Ctrl Pts',(2.63003080648701,-9.02673455434159,108.385444985715));
#46552=CARTESIAN_POINT('Ctrl Pts',(2.67461872355916,-9.02014529634552,108.507237281181));
#46553=CARTESIAN_POINT('Ctrl Pts',(2.78523979738068,-9.01355603834945,108.604854969331));
#46554=CARTESIAN_POINT('Ctrl Pts',(2.91163288575999,-9.00696678035337,108.633945050007));
#46555=CARTESIAN_POINT('Ctrl Pts',(3.0380259741393,-9.0003775223573,108.663035130683));
#46556=CARTESIAN_POINT('Ctrl Pts',(3.18019107707638,-8.99378826436123,108.623597603887));
#46557=CARTESIAN_POINT('Ctrl Pts',(3.27353489235059,-8.98719900636515,108.533551072949));
#46558=CARTESIAN_POINT('Ctrl Pts',(3.36687870762481,-8.98060974836908,108.443504542012));
#46559=CARTESIAN_POINT('Ctrl Pts',(3.41140123523617,-8.97402049037301,108.302849006934));
#46560=CARTESIAN_POINT('Ctrl Pts',(3.3868734807111,-8.96743123237693,108.175491891539));
#46561=CARTESIAN_POINT('Ctrl Pts',(3.36234572618602,-8.96084197438086,108.048134776144));
#46562=CARTESIAN_POINT('Ctrl Pts',(3.26876768952452,-8.95425271638479,107.934076080432));
#46563=CARTESIAN_POINT('Ctrl Pts',(3.14865693852936,-8.94766345838871,107.885138844311));
#46564=CARTESIAN_POINT('Ctrl Pts',(3.02854618753419,-8.94107420039264,107.836201608189));
#46565=CARTESIAN_POINT('Ctrl Pts',(2.88190272220536,-8.93448494239657,107.852385831659));
#46566=CARTESIAN_POINT('Ctrl Pts',(2.77535460722962,-8.92789568440049,107.926338145882));
#46567=CARTESIAN_POINT('Ctrl Pts',(2.67197818794736,-8.92150257366816,107.998089067461));
#46568=CARTESIAN_POINT('Ctrl Pts',(2.60634555296498,-8.91510946293583,108.124220019083));
#46569=CARTESIAN_POINT('Ctrl Pts',(2.60603291882732,-8.9087163522035,108.250070364255));
#46570=CARTESIAN_POINT('Ctrl Pts',(2.60603107819738,-8.8903836477965,108.250066160239));
#46571=CARTESIAN_POINT('Ctrl Pts',(2.60632683596882,-8.89678865363268,108.12398321277));
#46572=CARTESIAN_POINT('Ctrl Pts',(2.67223797731359,-8.90319365946885,107.997634228976));
#46573=CARTESIAN_POINT('Ctrl Pts',(2.77593552102208,-8.90959866530503,107.925935693686));
#46574=CARTESIAN_POINT('Ctrl Pts',(2.88261612156037,-8.9161879233011,107.85217461383));
#46575=CARTESIAN_POINT('Ctrl Pts',(3.02928838930142,-8.92277718129717,107.836253455542));
#46576=CARTESIAN_POINT('Ctrl Pts',(3.14931117306339,-8.92936643929325,107.885406062908));
#46577=CARTESIAN_POINT('Ctrl Pts',(3.26933395682536,-8.93595569728932,107.934558670273));
#46578=CARTESIAN_POINT('Ctrl Pts',(3.36270725660825,-8.94254495528539,108.048785043293));
#46579=CARTESIAN_POINT('Ctrl Pts',(3.38700652765649,-8.94913421328147,108.17618595718));
#46580=CARTESIAN_POINT('Ctrl Pts',(3.41130579870474,-8.95572347127754,108.303586871068));
#46581=CARTESIAN_POINT('Ctrl Pts',(3.36653104101834,-8.96231272927362,108.444162325823));
#46582=CARTESIAN_POINT('Ctrl Pts',(3.27302585084809,-8.96890198726969,108.534041282448));
#46583=CARTESIAN_POINT('Ctrl Pts',(3.17952066067784,-8.97549124526576,108.623920239073));
#46584=CARTESIAN_POINT('Ctrl Pts',(3.03728503802373,-8.98208050326183,108.663102697569));
#46585=CARTESIAN_POINT('Ctrl Pts',(2.91094432603153,-8.98866976125791,108.633785945939));
#46586=CARTESIAN_POINT('Ctrl Pts',(2.78460361403932,-8.99525901925398,108.604469194309));
#46587=CARTESIAN_POINT('Ctrl Pts',(2.67415781270903,-9.00184827725005,108.506653232554));
#46588=CARTESIAN_POINT('Ctrl Pts',(2.62978842845092,-9.00843753524613,108.384781147262));
#46589=CARTESIAN_POINT('Ctrl Pts',(2.61419766253913,-9.01075290609625,108.341957042652));
#46590=CARTESIAN_POINT('Ctrl Pts',(2.60676547676824,-9.01306827694638,108.296162682987));
#46591=CARTESIAN_POINT('Ctrl Pts',(2.60706396640167,-9.0153836477965,108.250274710706));
#46592=CARTESIAN_POINT('Origin',(3.,-8.675,108.25));
#46593=CARTESIAN_POINT('',(2.60697943945107,-9.1587163522035,108.24969186562));
#46594=CARTESIAN_POINT('',(2.60698518571652,-9.1403836477965,108.249693765459));
#46595=CARTESIAN_POINT('',(2.6067,-8.675,108.25));
#46596=CARTESIAN_POINT('Ctrl Pts',(2.60697943945107,-9.1587163522035,108.24969186562));
#46597=CARTESIAN_POINT('Ctrl Pts',(2.60763355898486,-9.1542579675593,108.338003969973));
#46598=CARTESIAN_POINT('Ctrl Pts',(2.63709990068649,-9.14979958291511,108.426711728349));
#46599=CARTESIAN_POINT('Ctrl Pts',(2.69175327539567,-9.14534119827092,108.495370138938));
#46600=CARTESIAN_POINT('Ctrl Pts',(2.77252808848497,-9.13875194027485,108.596843658403));
#46601=CARTESIAN_POINT('Ctrl Pts',(2.90831965608537,-9.13216268227877,108.654522815708));
#46602=CARTESIAN_POINT('Ctrl Pts',(3.03743051806054,-9.1255734242827,108.642200847298));
#46603=CARTESIAN_POINT('Ctrl Pts',(3.16654138003572,-9.11898416628663,108.629878878888));
#46604=CARTESIAN_POINT('Ctrl Pts',(3.28897153638567,-9.11239490829055,108.547555784765));
#46605=CARTESIAN_POINT('Ctrl Pts',(3.34909433947442,-9.10580565029448,108.432635403056));
#46606=CARTESIAN_POINT('Ctrl Pts',(3.40921714256317,-9.09921639229841,108.317715021347));
#46607=CARTESIAN_POINT('Ctrl Pts',(3.40703259239072,-9.09262713430233,108.170197352054));
#46608=CARTESIAN_POINT('Ctrl Pts',(3.34353324834952,-9.08603787630626,108.057107658049));
#46609=CARTESIAN_POINT('Ctrl Pts',(3.28003390430832,-9.07944861831018,107.944017964045));
#46610=CARTESIAN_POINT('Ctrl Pts',(3.15521976639838,-9.07285936031411,107.865356245329));
#46611=CARTESIAN_POINT('Ctrl Pts',(3.02580065415689,-9.06627010231804,107.856862778983));
#46612=CARTESIAN_POINT('Ctrl Pts',(2.8963815419154,-9.05968084432196,107.848369312637));
#46613=CARTESIAN_POINT('Ctrl Pts',(2.76235745534236,-9.05309158632589,107.910044098659));
#46614=CARTESIAN_POINT('Ctrl Pts',(2.68462279221722,-9.04650232832981,108.013864943062));
#46615=CARTESIAN_POINT('Ctrl Pts',(2.63434330462809,-9.04224033628771,108.081017210118));
#46616=CARTESIAN_POINT('Ctrl Pts',(2.60761317356649,-9.0379783442456,108.165801787015));
#46617=CARTESIAN_POINT('Ctrl Pts',(2.60706905675086,-9.03371635220349,108.250272277881));
#46618=CARTESIAN_POINT('Ctrl Pts',(2.60706396640167,-9.0153836477965,108.250274710706));
#46619=CARTESIAN_POINT('Ctrl Pts',(2.60761494120877,-9.01965753494245,108.165571210669));
#46620=CARTESIAN_POINT('Ctrl Pts',(2.63450631907698,-9.0239314220884,108.080548748322));
#46621=CARTESIAN_POINT('Ctrl Pts',(2.68504684679851,-9.02820530923435,108.013299605715));
#46622=CARTESIAN_POINT('Ctrl Pts',(2.76296761659014,-9.03479456723042,107.909618358289));
#46623=CARTESIAN_POINT('Ctrl Pts',(2.89710212335932,-9.0413838252265,107.848184072265));
#46624=CARTESIAN_POINT('Ctrl Pts',(3.02650579945226,-9.04797308322257,107.856909669463));
#46625=CARTESIAN_POINT('Ctrl Pts',(3.15590947554519,-9.05456234121864,107.865635266662));
#46626=CARTESIAN_POINT('Ctrl Pts',(3.28058232096189,-9.06115159921472,107.944520747083));
#46627=CARTESIAN_POINT('Ctrl Pts',(3.34387871299737,-9.06774085721079,108.05772416659));
#46628=CARTESIAN_POINT('Ctrl Pts',(3.40717510503286,-9.07433011520686,108.170927586097));
#46629=CARTESIAN_POINT('Ctrl Pts',(3.40909504368714,-9.08091937320294,108.31844894469));
#46630=CARTESIAN_POINT('Ctrl Pts',(3.34876619689658,-9.08750863119901,108.433261303248));
#46631=CARTESIAN_POINT('Ctrl Pts',(3.28843735010602,-9.09409788919509,108.548073661807));
#46632=CARTESIAN_POINT('Ctrl Pts',(3.16585971787063,-9.10068714719116,108.63017702033));
#46633=CARTESIAN_POINT('Ctrl Pts',(3.03672695412273,-9.10727640518723,108.642267378464));
#46634=CARTESIAN_POINT('Ctrl Pts',(2.90759419037484,-9.11386566318331,108.654357736598));
#46635=CARTESIAN_POINT('Ctrl Pts',(2.77190629511443,-9.12045492117938,108.596435094343));
#46636=CARTESIAN_POINT('Ctrl Pts',(2.69131362448212,-9.12704417917545,108.494816843654));
#46637=CARTESIAN_POINT('Ctrl Pts',(2.63692897795453,-9.1314906687158,108.426243949852));
#46638=CARTESIAN_POINT('Ctrl Pts',(2.60763287690707,-9.13593715825616,108.337773519252));
#46639=CARTESIAN_POINT('Ctrl Pts',(2.60698518571652,-9.1403836477965,108.249693765459));
#46640=CARTESIAN_POINT('Origin',(3.,-8.675,108.25));
#46641=CARTESIAN_POINT('',(2.60601707190308,-9.2837163522035,108.250000088186));
#46642=CARTESIAN_POINT('',(2.60601708531384,-9.26538364779651,108.249995786147));
#46643=CARTESIAN_POINT('',(2.6067,-8.675,108.25));
#46644=CARTESIAN_POINT('Ctrl Pts',(2.60601707359714,-9.2837163522035,108.250000088186));
#46645=CARTESIAN_POINT('Ctrl Pts',(2.60601663870951,-9.27712684886908,108.379702432267));
#46646=CARTESIAN_POINT('Ctrl Pts',(2.67634181801385,-9.27053734553466,108.509404370714));
#46647=CARTESIAN_POINT('Ctrl Pts',(2.78503705730119,-9.26394784220024,108.580171898013));
#46648=CARTESIAN_POINT('Ctrl Pts',(2.8937282496811,-9.25735858420417,108.650936790518));
#46649=CARTESIAN_POINT('Ctrl Pts',(3.04078664484427,-9.2507693262081,108.662771660248));
#46650=CARTESIAN_POINT('Ctrl Pts',(3.15939564839677,-9.24418006821202,108.610299286235));
#46651=CARTESIAN_POINT('Ctrl Pts',(3.27800465194927,-9.23759081021595,108.557826912222));
#46652=CARTESIAN_POINT('Ctrl Pts',(3.36816426389111,-9.23100155221988,108.441047294465));
#46653=CARTESIAN_POINT('Ctrl Pts',(3.38891009394621,-9.2244122942238,108.313019734585));
#46654=CARTESIAN_POINT('Ctrl Pts',(3.40965592400131,-9.21782303622773,108.184992174704));
#46655=CARTESIAN_POINT('Ctrl Pts',(3.36098797216966,-9.21123377823166,108.045716672699));
#46656=CARTESIAN_POINT('Ctrl Pts',(3.26501872258032,-9.20464452023558,107.958473628877));
#46657=CARTESIAN_POINT('Ctrl Pts',(3.16904947299098,-9.19805526223951,107.871230585055));
#46658=CARTESIAN_POINT('Ctrl Pts',(3.02577892564394,-9.19146600424344,107.836019999416));
#46659=CARTESIAN_POINT('Ctrl Pts',(2.90030264644593,-9.18487674624736,107.868839947004));
#46660=CARTESIAN_POINT('Ctrl Pts',(2.77482636724793,-9.17828748825129,107.901659894592));
#46661=CARTESIAN_POINT('Ctrl Pts',(2.66714435619896,-9.17169823025521,108.002510375407));
#46662=CARTESIAN_POINT('Ctrl Pts',(2.62618237996357,-9.16510897225914,108.125569556628));
#46663=CARTESIAN_POINT('Ctrl Pts',(2.61293585301738,-9.16297809890726,108.165365164892));
#46664=CARTESIAN_POINT('Ctrl Pts',(2.60666680472018,-9.16084722555538,108.207483324896));
#46665=CARTESIAN_POINT('Ctrl Pts',(2.60697943945107,-9.1587163522035,108.24969186562));
#46666=CARTESIAN_POINT('Ctrl Pts',(2.60698518571652,-9.1403836477965,108.249693765459));
#46667=CARTESIAN_POINT('Ctrl Pts',(2.60667306258218,-9.14252641625223,108.207248030166));
#46668=CARTESIAN_POINT('Ctrl Pts',(2.61301392315575,-9.14466918470795,108.16489302125));
#46669=CARTESIAN_POINT('Ctrl Pts',(2.62640615645749,-9.14681195316367,108.1248992189));
#46670=CARTESIAN_POINT('Ctrl Pts',(2.66758880506941,-9.15340121115974,108.001913703958));
#46671=CARTESIAN_POINT('Ctrl Pts',(2.77545154829749,-9.15999046915582,107.901256533195));
#46672=CARTESIAN_POINT('Ctrl Pts',(2.90098650287746,-9.16657972715189,107.868661708252));
#46673=CARTESIAN_POINT('Ctrl Pts',(3.02652145745744,-9.17316898514797,107.836066883309));
#46674=CARTESIAN_POINT('Ctrl Pts',(3.1697286233893,-9.17975824314404,107.871534404184));
#46675=CARTESIAN_POINT('Ctrl Pts',(3.2655412327813,-9.18634750114011,107.958949456164));
#46676=CARTESIAN_POINT('Ctrl Pts',(3.3613538421733,-9.19293675913618,108.046364508145));
#46677=CARTESIAN_POINT('Ctrl Pts',(3.40977189502544,-9.19952601713226,108.18572709123));
#46678=CARTESIAN_POINT('Ctrl Pts',(3.38879644895739,-9.20611527512833,108.313717239644));
#46679=CARTESIAN_POINT('Ctrl Pts',(3.36782100288935,-9.21270453312441,108.441707388058));
#46680=CARTESIAN_POINT('Ctrl Pts',(3.27745205790112,-9.21929379112049,108.5583251018));
#46681=CARTESIAN_POINT('Ctrl Pts',(3.15874911753129,-9.22588304911656,108.61058464062));
#46682=CARTESIAN_POINT('Ctrl Pts',(3.04004617716147,-9.23247230711263,108.662844179439));
#46683=CARTESIAN_POINT('Ctrl Pts',(2.89300924141004,-9.2390615651087,108.650745543336));
#46684=CARTESIAN_POINT('Ctrl Pts',(2.78444515030389,-9.24565082310478,108.57978579747));
#46685=CARTESIAN_POINT('Ctrl Pts',(2.6760729998083,-9.25222843133535,108.508951507975));
#46686=CARTESIAN_POINT('Ctrl Pts',(2.6060377747357,-9.25880603956593,108.379464056852));
#46687=CARTESIAN_POINT('Ctrl Pts',(2.60601710832407,-9.26538364779651,108.249995786289));
#46688=CARTESIAN_POINT('Origin',(3.,-8.675,108.25));
#46689=CARTESIAN_POINT('',(2.60697942739454,-9.4087163522035,108.250308115953));
#46690=CARTESIAN_POINT('',(2.60697382714618,-9.3903836477965,108.250309930203));
#46691=CARTESIAN_POINT('',(2.6067,-8.675,108.25));
#46692=CARTESIAN_POINT('Ctrl Pts',(2.60697942739454,-9.4087163522035,108.250308115953));
#46693=CARTESIAN_POINT('Ctrl Pts',(2.60666701491607,-9.40658498817493,108.292526395753));
#46694=CARTESIAN_POINT('Ctrl Pts',(2.61293922160114,-9.40445362414636,108.334654279803));
#46695=CARTESIAN_POINT('Ctrl Pts',(2.62619185344577,-9.40232226011779,108.374458046898));
#46696=CARTESIAN_POINT('Ctrl Pts',(2.66716327324111,-9.39573300212172,108.497514121361));
#46697=CARTESIAN_POINT('Ctrl Pts',(2.7748521733323,-9.38914374412564,108.598356759879));
#46698=CARTESIAN_POINT('Ctrl Pts',(2.90033072587369,-9.38255448612957,108.631167456806));
#46699=CARTESIAN_POINT('Ctrl Pts',(3.02580927841509,-9.3759652281335,108.663978153734));
#46700=CARTESIAN_POINT('Ctrl Pts',(3.16907748340668,-9.36937597013742,108.628756909072));
#46701=CARTESIAN_POINT('Ctrl Pts',(3.26504034884136,-9.36278671214135,108.541506748758));
#46702=CARTESIAN_POINT('Ctrl Pts',(3.36100321427603,-9.35619745414527,108.454256588444));
#46703=CARTESIAN_POINT('Ctrl Pts',(3.40966074015377,-9.3496081961492,108.314977512479));
#46704=CARTESIAN_POINT('Ctrl Pts',(3.38890540409867,-9.34301893815313,108.186951495083));
#46705=CARTESIAN_POINT('Ctrl Pts',(3.36815006804357,-9.33642968015705,108.058925477687));
#46706=CARTESIAN_POINT('Ctrl Pts',(3.27798187005562,-9.32984042216098,107.94215251886));
#46707=CARTESIAN_POINT('Ctrl Pts',(3.15936899998641,-9.32325116416491,107.889688917974));
#46708=CARTESIAN_POINT('Ctrl Pts',(3.04075612991719,-9.31666190616883,107.837225317089));
#46709=CARTESIAN_POINT('Ctrl Pts',(2.8936985877667,-9.31007264817276,107.849071074143));
#46710=CARTESIAN_POINT('Ctrl Pts',(2.78501262337676,-9.30348339017669,107.919844009963));
#46711=CARTESIAN_POINT('Ctrl Pts',(2.67633070569959,-9.29689437751896,107.990614310688));
#46712=CARTESIAN_POINT('Ctrl Pts',(2.6060175084524,-9.29030536486123,108.12030740218));
#46713=CARTESIAN_POINT('Ctrl Pts',(2.60601707359714,-9.2837163522035,108.250000088186));
#46714=CARTESIAN_POINT('Ctrl Pts',(2.60601710832407,-9.26538364779651,108.249995786289));
#46715=CARTESIAN_POINT('Ctrl Pts',(2.60599636870685,-9.27198455555808,108.120068906779));
#46716=CARTESIAN_POINT('Ctrl Pts',(2.67660005833137,-9.27858546331965,107.990161542424));
#46717=CARTESIAN_POINT('Ctrl Pts',(2.78560517593341,-9.28518637108122,107.919458890809));
#46718=CARTESIAN_POINT('Ctrl Pts',(2.89441791331987,-9.29177562907729,107.848881020413));
#46719=CARTESIAN_POINT('Ctrl Pts',(3.04149645195734,-9.29836488707337,107.837299069189));
#46720=CARTESIAN_POINT('Ctrl Pts',(3.16001504540131,-9.30495414506944,107.889975346291));
#46721=CARTESIAN_POINT('Ctrl Pts',(3.27853363884528,-9.31154340306551,107.942651623393));
#46722=CARTESIAN_POINT('Ctrl Pts',(3.36849228709577,-9.31813266106159,108.05958612882));
#46723=CARTESIAN_POINT('Ctrl Pts',(3.38901791601593,-9.32472191905766,108.187649182856));
#46724=CARTESIAN_POINT('Ctrl Pts',(3.40954354493609,-9.33131117705373,108.315712236891));
#46725=CARTESIAN_POINT('Ctrl Pts',(3.36063615452594,-9.33790043504981,108.454903839535));
#46726=CARTESIAN_POINT('Ctrl Pts',(3.26451699895289,-9.34448969304588,108.541981718934));
#46727=CARTESIAN_POINT('Ctrl Pts',(3.16839784337984,-9.35107895104196,108.629059598332));
#46728=CARTESIAN_POINT('Ctrl Pts',(3.0250669226439,-9.35766820903803,108.664023754484));
#46729=CARTESIAN_POINT('Ctrl Pts',(2.89964727847269,-9.3642574670341,108.630988060613));
#46730=CARTESIAN_POINT('Ctrl Pts',(2.77422763430147,-9.37084672503017,108.597952366742));
#46731=CARTESIAN_POINT('Ctrl Pts',(2.66671926669498,-9.37743598302625,108.496916822849));
#46732=CARTESIAN_POINT('Ctrl Pts',(2.62596894818531,-9.38402524102232,108.373787384875));
#46733=CARTESIAN_POINT('Ctrl Pts',(2.61286139741018,-9.38614470994705,108.334182164127));
#46734=CARTESIAN_POINT('Ctrl Pts',(2.60666077129626,-9.38826417887178,108.292291063789));
#46735=CARTESIAN_POINT('Ctrl Pts',(2.60697382714618,-9.3903836477965,108.250309930203));
#46736=CARTESIAN_POINT('Origin',(3.,-8.675,108.25));
#46737=CARTESIAN_POINT('',(2.60697877099099,-9.5337163522035,108.249759674367));
#46738=CARTESIAN_POINT('',(2.60706672186757,-9.51538364779651,108.249732606859));
#46739=CARTESIAN_POINT('',(2.6067,-8.675,108.25));
#46740=CARTESIAN_POINT('Ctrl Pts',(2.60697877099099,-9.5337163522035,108.249759674367));
#46741=CARTESIAN_POINT('Ctrl Pts',(2.60754699255653,-9.52945386948471,108.334231172059));
#46742=CARTESIAN_POINT('Ctrl Pts',(2.63434920343294,-9.52519138676591,108.419009166244));
#46743=CARTESIAN_POINT('Ctrl Pts',(2.68466392975194,-9.52092890404712,108.486158593116));
#46744=CARTESIAN_POINT('Ctrl Pts',(2.762444119043,-9.51433964605104,108.589963095596));
#46745=CARTESIAN_POINT('Ctrl Pts',(2.89641273295953,-9.50775038805497,108.651640186054));
#46746=CARTESIAN_POINT('Ctrl Pts',(3.02581531647536,-9.50116113005889,108.643140007765));
#46747=CARTESIAN_POINT('Ctrl Pts',(3.1552178999912,-9.49457187206282,108.634639829476));
#46748=CARTESIAN_POINT('Ctrl Pts',(3.28005445310634,-9.48798261406675,108.555962382439));
#46749=CARTESIAN_POINT('Ctrl Pts',(3.3435531514507,-9.48139335607067,108.442866111883));
#46750=CARTESIAN_POINT('Ctrl Pts',(3.40705184979507,-9.4748040980746,108.329769841328));
#46751=CARTESIAN_POINT('Ctrl Pts',(3.40921269336866,-9.46821484007852,108.182254747253));
#46752=CARTESIAN_POINT('Ctrl Pts',(3.34907795614323,-9.46162558208245,108.067339519195));
#46753=CARTESIAN_POINT('Ctrl Pts',(3.2889432189178,-9.45503632408638,107.952424291138));
#46754=CARTESIAN_POINT('Ctrl Pts',(3.16651290089336,-9.4484470660903,107.870108929098));
#46755=CARTESIAN_POINT('Ctrl Pts',(3.03740273717822,-9.44185780809423,107.857796145506));
#46756=CARTESIAN_POINT('Ctrl Pts',(2.90829257346308,-9.43526855009816,107.845483361913));
#46757=CARTESIAN_POINT('Ctrl Pts',(2.77250256405724,-9.42867929210209,107.903173156768));
#46758=CARTESIAN_POINT('Ctrl Pts',(2.69173452910408,-9.42209003410601,108.004652809398));
#46759=CARTESIAN_POINT('Ctrl Pts',(2.63709175506193,-9.41763214013851,108.073307812975));
#46760=CARTESIAN_POINT('Ctrl Pts',(2.60763285950868,-9.413174246171,108.162005689753));
#46761=CARTESIAN_POINT('Ctrl Pts',(2.60697942739454,-9.4087163522035,108.250308115953));
#46762=CARTESIAN_POINT('Ctrl Pts',(2.60697382714618,-9.3903836477965,108.250309930203));
#46763=CARTESIAN_POINT('Ctrl Pts',(2.60763403669223,-9.39485343686785,108.161775104372));
#46764=CARTESIAN_POINT('Ctrl Pts',(2.63726411326604,-9.3993232259392,108.072839851989));
#46765=CARTESIAN_POINT('Ctrl Pts',(2.69217563494894,-9.40379301501054,108.004100125204));
#46766=CARTESIAN_POINT('Ctrl Pts',(2.77312490963509,-9.41038227300661,107.902765635559));
#46767=CARTESIAN_POINT('Ctrl Pts',(2.90901572842025,-9.41697153100269,107.845319988321));
#46768=CARTESIAN_POINT('Ctrl Pts',(3.03810506853297,-9.42356078899876,107.857864034878));
#46769=CARTESIAN_POINT('Ctrl Pts',(3.1671944086457,-9.43015004699484,107.870408081435));
#46770=CARTESIAN_POINT('Ctrl Pts',(3.28948227008599,-9.43673930499091,107.952941821786));
#46771=CARTESIAN_POINT('Ctrl Pts',(3.34940767562958,-9.44332856298699,108.067965307736));
#46772=CARTESIAN_POINT('Ctrl Pts',(3.40933308117317,-9.44991782098306,108.182988793687));
#46773=CARTESIAN_POINT('Ctrl Pts',(3.40689603082006,-9.45650707897913,108.330502025238));
#46774=CARTESIAN_POINT('Ctrl Pts',(3.34320159534457,-9.46309633697521,108.443482625721));
#46775=CARTESIAN_POINT('Ctrl Pts',(3.27950715986907,-9.46968559497128,108.556463226204));
#46776=CARTESIAN_POINT('Ctrl Pts',(3.15455533927118,-9.47627485296735,108.634911195619));
#46777=CARTESIAN_POINT('Ctrl Pts',(3.0251233356586,-9.48286411096342,108.643181463371));
#46778=CARTESIAN_POINT('Ctrl Pts',(2.89569133204601,-9.4894533689595,108.651451731123));
#46779=CARTESIAN_POINT('Ctrl Pts',(2.76177914541873,-9.49604262695558,108.589544297211));
#46780=CARTESIAN_POINT('Ctrl Pts',(2.68421986242852,-9.50263188495165,108.485591155156));
#46781=CARTESIAN_POINT('Ctrl Pts',(2.6341880488466,-9.5068824725666,108.418533234762));
#46782=CARTESIAN_POINT('Ctrl Pts',(2.60760614734699,-9.51113306018155,108.333978999258));
#46783=CARTESIAN_POINT('Ctrl Pts',(2.60706672186757,-9.51538364779651,108.249732606859));
#46784=CARTESIAN_POINT('Origin',(3.,-7.51222265507269,108.25));
#46785=CARTESIAN_POINT('',(2.67795342847984,-9.57472265507269,108.249803074133));
#46786=CARTESIAN_POINT('',(2.67772883664542,-9.59937734492731,108.249997529819));
#46787=CARTESIAN_POINT('',(2.677725,-7.51222265507269,108.25));
#46788=CARTESIAN_POINT('',(2.90469398989908,-9.6,107.942139739389));
#46789=CARTESIAN_POINT('Ctrl Pts',(2.67795342847984,-9.57472265507269,108.249803074133));
#46790=CARTESIAN_POINT('Ctrl Pts',(2.67769926555923,-9.57704943034997,108.212019357596));
#46791=CARTESIAN_POINT('Ctrl Pts',(2.69997452530982,-9.58547521199241,108.07546693902));
#46792=CARTESIAN_POINT('Ctrl Pts',(2.81100303866955,-9.59390099363485,107.971242620752));
#46793=CARTESIAN_POINT('Ctrl Pts',(2.90476631137571,-9.6,107.941669514675));
#46794=CARTESIAN_POINT('',(2.67788283232033,-9.6,108.239915065145));
#46795=CARTESIAN_POINT('Origin',(3.,-9.6,108.25));
#46796=CARTESIAN_POINT('Ctrl Pts',(2.67772883664542,-9.59937734492731,108.249997529819));
#46797=CARTESIAN_POINT('Ctrl Pts',(2.67772642548982,-9.59958489661821,108.246636930255));
#46798=CARTESIAN_POINT('Ctrl Pts',(2.67777761936289,-9.5997924483091,108.243275612371));
#46799=CARTESIAN_POINT('Ctrl Pts',(2.67788283232033,-9.6,108.239915065145));
#46800=CARTESIAN_POINT('Origin',(3.,-7.51222265507269,108.25));
#46801=CARTESIAN_POINT('',(2.67795396634523,-9.44972265507269,108.250252474113));
#46802=CARTESIAN_POINT('',(2.67802549654176,-9.47437734492731,108.249780894675));
#46803=CARTESIAN_POINT('',(2.677725,-7.51222265507269,108.25));
#46804=CARTESIAN_POINT('Ctrl Pts',(2.67795396634523,-9.44972265507269,108.250252474113));
#46805=CARTESIAN_POINT('Ctrl Pts',(2.67848939689337,-9.4541805490402,108.177896347992));
#46806=CARTESIAN_POINT('Ctrl Pts',(2.73830847628814,-9.46522770100378,107.997786902831));
#46807=CARTESIAN_POINT('Ctrl Pts',(3.03612182658042,-9.48286411096343,107.871262196348));
#46808=CARTESIAN_POINT('Ctrl Pts',(3.33708468501923,-9.50263188495165,108.073612946168));
#46809=CARTESIAN_POINT('Ctrl Pts',(3.33177281726424,-9.52239965893987,108.436240153971));
#46810=CARTESIAN_POINT('Ctrl Pts',(3.02489486032158,-9.54216743292809,108.629648042939));
#46811=CARTESIAN_POINT('Ctrl Pts',(2.73433168531756,-9.55960843163903,108.495877223755));
#46812=CARTESIAN_POINT('Ctrl Pts',(2.67841903642552,-9.5704601723539,108.319020088928));
#46813=CARTESIAN_POINT('Ctrl Pts',(2.67795342847984,-9.57472265507269,108.249803074133));
#46814=CARTESIAN_POINT('Ctrl Pts',(2.67802549654176,-9.47437734492731,108.249780894675));
#46815=CARTESIAN_POINT('Ctrl Pts',(2.67778230180603,-9.47671601530843,108.211799227294));
#46816=CARTESIAN_POINT('Ctrl Pts',(2.701514674746,-9.48564394368563,108.067094842141));
#46817=CARTESIAN_POINT('Ctrl Pts',(2.91535037624978,-9.50116113005889,107.879072987278));
#46818=CARTESIAN_POINT('Ctrl Pts',(3.26451785003709,-9.52092890404712,107.976673691963));
#46819=CARTESIAN_POINT('Ctrl Pts',(3.37368648223413,-9.54069667803533,108.322492331795));
#46820=CARTESIAN_POINT('Ctrl Pts',(3.1425103302508,-9.56046445202356,108.602707172509));
#46821=CARTESIAN_POINT('Ctrl Pts',(2.84350450152926,-9.57693759701374,108.568400494187));
#46822=CARTESIAN_POINT('Ctrl Pts',(2.7023541417074,-9.58990856131499,108.402984030974));
#46823=CARTESIAN_POINT('Ctrl Pts',(2.67776469963313,-9.59629026762017,108.299982334113));
#46824=CARTESIAN_POINT('Ctrl Pts',(2.67772883664542,-9.59937734492731,108.249997529819));
#46825=CARTESIAN_POINT('Origin',(3.,-7.51222265507269,108.25));
#46826=CARTESIAN_POINT('',(2.677165376484,-9.32472265507269,108.250000072264));
#46827=CARTESIAN_POINT('',(2.6779493774308,-9.34937734492731,108.250253960733));
#46828=CARTESIAN_POINT('',(2.677725,-7.51222265507269,108.25));
#46829=CARTESIAN_POINT('Ctrl Pts',(2.67716540145823,-9.32472265507269,108.250000072261));
#46830=CARTESIAN_POINT('Ctrl Pts',(2.67716575778413,-9.33131166773042,108.143728243167));
#46831=CARTESIAN_POINT('Ctrl Pts',(2.79239895133995,-9.34448993838423,107.931179963473));
#46832=CARTESIAN_POINT('Ctrl Pts',(3.15389690100588,-9.3642574670341,107.902060634909));
#46833=CARTESIAN_POINT('Ctrl Pts',(3.37555179045336,-9.38402524102232,108.189116358066));
#46834=CARTESIAN_POINT('Ctrl Pts',(3.25594001202276,-9.40379301501054,108.531497473297));
#46835=CARTESIAN_POINT('Ctrl Pts',(2.9037526682877,-9.42356078899877,108.618079674849));
#46836=CARTESIAN_POINT('Ctrl Pts',(2.69872669280949,-9.43887066901948,108.426088111054));
#46837=CARTESIAN_POINT('Ctrl Pts',(2.67769797160457,-9.44759129104412,108.284846667153));
#46838=CARTESIAN_POINT('Ctrl Pts',(2.67795396634523,-9.44972265507269,108.250252474113));
#46839=CARTESIAN_POINT('Ctrl Pts',(2.6779493774308,-9.34937734492731,108.250253960733));
#46840=CARTESIAN_POINT('Ctrl Pts',(2.67849036149248,-9.35384713399866,108.177707403411));
#46841=CARTESIAN_POINT('Ctrl Pts',(2.73856153576217,-9.36490618106608,107.997402602939));
#46842=CARTESIAN_POINT('Ctrl Pts',(3.03679699339086,-9.38255448612957,107.871328383607));
#46843=CARTESIAN_POINT('Ctrl Pts',(3.3374096596431,-9.40232226011779,108.074215959287));
#46844=CARTESIAN_POINT('Ctrl Pts',(3.33141880989063,-9.42209003410602,108.436838588562));
#46845=CARTESIAN_POINT('Ctrl Pts',(3.0242574980433,-9.44185780809423,108.629682366924));
#46846=CARTESIAN_POINT('Ctrl Pts',(2.73401479394391,-9.45928691170134,108.495503533206));
#46847=CARTESIAN_POINT('Ctrl Pts',(2.67846750860984,-9.47012675731236,108.318813455342));
#46848=CARTESIAN_POINT('Ctrl Pts',(2.67802549654176,-9.47437734492731,108.249780894675));
#46849=CARTESIAN_POINT('Origin',(3.,-7.51222265507269,108.25));
#46850=CARTESIAN_POINT('',(2.6779539762245,-9.19972265507269,108.249747510787));
#46851=CARTESIAN_POINT('',(2.67716540814336,-9.22437734492731,108.249996547097));
#46852=CARTESIAN_POINT('',(2.677725,-7.51222265507269,108.25));
#46853=CARTESIAN_POINT('Ctrl Pts',(2.6779539762245,-9.19972265507269,108.249747510787));
#46854=CARTESIAN_POINT('Ctrl Pts',(2.67769779936739,-9.20185352842457,108.21516129807));
#46855=CARTESIAN_POINT('Ctrl Pts',(2.69871958846501,-9.21057365977253,108.073927886744));
#46856=CARTESIAN_POINT('Ctrl Pts',(2.90372587748699,-9.22588304911656,107.881927545957));
#46857=CARTESIAN_POINT('Ctrl Pts',(3.25591897928919,-9.24565082310478,107.968483545095));
#46858=CARTESIAN_POINT('Ctrl Pts',(3.37555638719568,-9.265418597093,108.310855874679));
#46859=CARTESIAN_POINT('Ctrl Pts',(3.15392260429289,-9.28518637108122,108.597927967071));
#46860=CARTESIAN_POINT('Ctrl Pts',(2.79241807110289,-9.30495414506944,108.568835040736));
#46861=CARTESIAN_POINT('Ctrl Pts',(2.67716719052207,-9.31813290639993,108.356283772265));
#46862=CARTESIAN_POINT('Ctrl Pts',(2.67716540144496,-9.32472240973435,108.250004029235));
#46863=CARTESIAN_POINT('Ctrl Pts',(2.67716540145823,-9.32472265507269,108.250000072261));
#46864=CARTESIAN_POINT('Ctrl Pts',(2.67716542991391,-9.22437734492731,108.249996547232));
#46865=CARTESIAN_POINT('Ctrl Pts',(2.67716539992112,-9.22438899469281,108.249808652243));
#46866=CARTESIAN_POINT('Ctrl Pts',(2.67725037642591,-9.23098990245438,108.143344949962));
#46867=CARTESIAN_POINT('Ctrl Pts',(2.7929666844032,-9.24418006821203,107.930808426606));
#46868=CARTESIAN_POINT('Ctrl Pts',(3.15452073504689,-9.26394784220025,107.902337234153));
#46869=CARTESIAN_POINT('Ctrl Pts',(3.37566050136972,-9.28371561618847,108.1897900773));
#46870=CARTESIAN_POINT('Ctrl Pts',(3.25543449645413,-9.30348339017669,108.531956162289));
#46871=CARTESIAN_POINT('Ctrl Pts',(2.90309298249399,-9.32325116416491,108.617906379101));
#46872=CARTESIAN_POINT('Ctrl Pts',(2.6985697470388,-9.33854914908178,108.42569700235));
#46873=CARTESIAN_POINT('Ctrl Pts',(2.67769285550344,-9.34725787600258,108.284653833162));
#46874=CARTESIAN_POINT('Ctrl Pts',(2.6779493774308,-9.34937734492731,108.250253960733));
#46875=CARTESIAN_POINT('Origin',(3.,-7.51222265507269,108.25));
#46876=CARTESIAN_POINT('',(2.67802740977468,-9.07472265507269,108.250223107943));
#46877=CARTESIAN_POINT('',(2.67795868478717,-9.09937734492731,108.24974906754));
#46878=CARTESIAN_POINT('',(2.677725,-7.51222265507269,108.25));
#46879=CARTESIAN_POINT('Ctrl Pts',(2.67802740977468,-9.07472265507269,108.250223107943));
#46880=CARTESIAN_POINT('Ctrl Pts',(2.67847326598307,-9.0789846471148,108.181006918155));
#46881=CARTESIAN_POINT('Ctrl Pts',(2.73423944584299,-9.08983589715298,108.004123686505));
#46882=CARTESIAN_POINT('Ctrl Pts',(3.02491475698223,-9.10727640518723,107.870361628692));
#46883=CARTESIAN_POINT('Ctrl Pts',(3.331737612016,-9.12704417917545,108.063730853703));
#46884=CARTESIAN_POINT('Ctrl Pts',(3.33710775623283,-9.14681195316367,108.426364392007));
#46885=CARTESIAN_POINT('Ctrl Pts',(3.0361452952284,-9.1665797271519,108.628734149129));
#46886=CARTESIAN_POINT('Ctrl Pts',(2.73832024171984,-9.18421662778823,108.502229253324));
#46887=CARTESIAN_POINT('Ctrl Pts',(2.678489970053,-9.1952642704285,108.32211156731));
#46888=CARTESIAN_POINT('Ctrl Pts',(2.6779539762245,-9.19972265507269,108.249747510787));
#46889=CARTESIAN_POINT('Ctrl Pts',(2.67795868478717,-9.09937734492731,108.24974906754));
#46890=CARTESIAN_POINT('Ctrl Pts',(2.67770292713876,-9.10152011338304,108.214968494589));
#46891=CARTESIAN_POINT('Ctrl Pts',(2.69887633057988,-9.11025213983483,108.073536636701));
#46892=CARTESIAN_POINT('Ctrl Pts',(2.90438625299112,-9.1255734242827,107.881755427227));
#46893=CARTESIAN_POINT('Ctrl Pts',(3.2564235481909,-9.14534119827092,107.968943034321));
#46894=CARTESIAN_POINT('Ctrl Pts',(3.37544664493324,-9.16510897225914,108.311529429926));
#46895=CARTESIAN_POINT('Ctrl Pts',(3.15329827158403,-9.18487674624737,108.59820352372));
#46896=CARTESIAN_POINT('Ctrl Pts',(2.79205950553832,-9.20463287047008,108.568479724359));
#46897=CARTESIAN_POINT('Ctrl Pts',(2.67718236423328,-9.21779973669674,108.35608448747));
#46898=CARTESIAN_POINT('Ctrl Pts',(2.67716542991391,-9.22437734492731,108.249996547232));
#46899=CARTESIAN_POINT('Origin',(3.,-7.51222265507269,108.25));
#46900=CARTESIAN_POINT('',(2.67717838524047,-8.94972265507269,108.250057657362));
#46901=CARTESIAN_POINT('',(2.67802323867811,-8.97437734492731,108.25022510143));
#46902=CARTESIAN_POINT('',(2.677725,-7.51222265507269,108.25));
#46903=CARTESIAN_POINT('Ctrl Pts',(2.67717838524047,-8.94972265507269,108.250057657362));
#46904=CARTESIAN_POINT('Ctrl Pts',(2.67743456161147,-8.95611576580502,108.146934290999));
#46905=CARTESIAN_POINT('Ctrl Pts',(2.78664501856536,-8.96909813453343,107.937056706984));
#46906=CARTESIAN_POINT('Ctrl Pts',(3.14355261982312,-8.9886697612579,107.897666800561));
#46907=CARTESIAN_POINT('Ctrl Pts',(3.37358970422498,-9.00843753524613,108.178050219025));
#46908=CARTESIAN_POINT('Ctrl Pts',(3.26414273560599,-9.02820530923435,108.523814998333));
#46909=CARTESIAN_POINT('Ctrl Pts',(2.91466707924407,-9.04797308322257,108.620761824788));
#46910=CARTESIAN_POINT('Ctrl Pts',(2.70136371725896,-9.06347886516868,108.432532038618));
#46911=CARTESIAN_POINT('Ctrl Pts',(2.67778394944817,-9.07239538911873,108.288018692817));
#46912=CARTESIAN_POINT('Ctrl Pts',(2.67802740977468,-9.07472265507269,108.250223107943));
#46913=CARTESIAN_POINT('Ctrl Pts',(2.67802323867811,-8.97437734492731,108.25022510143));
#46914=CARTESIAN_POINT('Ctrl Pts',(2.67847471441155,-8.97865123207326,108.180817980977));
#46915=CARTESIAN_POINT('Ctrl Pts',(2.73448248140951,-8.98951437721528,108.003738238763));
#46916=CARTESIAN_POINT('Ctrl Pts',(3.02559569024832,-9.00696678035338,107.87040690913));
#46917=CARTESIAN_POINT('Ctrl Pts',(3.332071214708,-9.02673455434159,108.064326193666));
#46918=CARTESIAN_POINT('Ctrl Pts',(3.33679088083925,-9.04650232832982,108.426968801146));
#46919=CARTESIAN_POINT('Ctrl Pts',(3.03546588901117,-9.06627010231804,108.628798395868));
#46920=CARTESIAN_POINT('Ctrl Pts',(2.73806892801327,-9.08389510785053,108.501845156991));
#46921=CARTESIAN_POINT('Ctrl Pts',(2.67848941114982,-9.09493085538696,108.321922733071));
#46922=CARTESIAN_POINT('Ctrl Pts',(2.67795868478717,-9.09937734492731,108.24974906754));
#46923=CARTESIAN_POINT('Origin',(3.,-7.51222265507269,108.25));
#46924=CARTESIAN_POINT('',(2.67787169029203,-8.82472265507269,108.249726345659));
#46925=CARTESIAN_POINT('',(2.67717687700499,-8.84937734492731,108.250054212538));
#46926=CARTESIAN_POINT('',(2.677725,-7.51222265507269,108.25));
#46927=CARTESIAN_POINT('Ctrl Pts',(2.67787169029203,-8.82472265507269,108.249726345659));
#46928=CARTESIAN_POINT('Ctrl Pts',(2.67761485306344,-8.82665762649918,108.218340113235));
#46929=CARTESIAN_POINT('Ctrl Pts',(2.69619998288975,-8.83518185592173,108.080370347943));
#46930=CARTESIAN_POINT('Ctrl Pts',(2.89289612067176,-8.85029534334036,107.884931791143));
#46931=CARTESIAN_POINT('Ctrl Pts',(3.24749216158505,-8.87006311732858,107.961047290999));
#46932=CARTESIAN_POINT('Ctrl Pts',(3.37719002903275,-8.88983089131681,108.299736506548));
#46933=CARTESIAN_POINT('Ctrl Pts',(3.16413219853988,-8.90959866530502,108.593229747382));
#46934=CARTESIAN_POINT('Ctrl Pts',(2.80192608220999,-8.92936643929325,108.574827278991));
#46935=CARTESIAN_POINT('Ctrl Pts',(2.67864156962831,-8.94274110254913,108.362665331578));
#46936=CARTESIAN_POINT('Ctrl Pts',(2.67717052548388,-8.94952650780894,108.253221589129));
#46937=CARTESIAN_POINT('Ctrl Pts',(2.67717838524047,-8.94972265507269,108.250057657362));
#46938=CARTESIAN_POINT('Ctrl Pts',(2.67717687700499,-8.84937734492731,108.250054212538));
#46939=CARTESIAN_POINT('Ctrl Pts',(2.67741922466783,-8.85578235076348,108.146740248908));
#46940=CARTESIAN_POINT('Ctrl Pts',(2.78698972715461,-8.86877661459573,107.936698041163));
#46941=CARTESIAN_POINT('Ctrl Pts',(3.14418439041029,-8.88836013642405,107.897924843879));
#46942=CARTESIAN_POINT('Ctrl Pts',(3.37371818283995,-8.90812791041227,108.178720453069));
#46943=CARTESIAN_POINT('Ctrl Pts',(3.26365117266921,-8.9278956844005,108.524288375886));
#46944=CARTESIAN_POINT('Ctrl Pts',(2.91400216206011,-8.94766345838871,108.620608183754));
#46945=CARTESIAN_POINT('Ctrl Pts',(2.70120014077517,-8.96315734523099,108.432140771461));
#46946=CARTESIAN_POINT('Ctrl Pts',(2.67777865249297,-8.97206197407719,108.287826286956));
#46947=CARTESIAN_POINT('Ctrl Pts',(2.67802323867811,-8.97437734492731,108.25022510143));
#46948=CARTESIAN_POINT('Origin',(3.,-7.51222265507269,108.25));
#46949=CARTESIAN_POINT('',(2.67808974459385,-8.69972265507269,108.25018671496));
#46950=CARTESIAN_POINT('',(2.67787688739042,-8.72437734492731,108.249727382091));
#46951=CARTESIAN_POINT('',(2.677725,-7.51222265507269,108.25));
#46952=CARTESIAN_POINT('Ctrl Pts',(2.67808974459385,-8.69972265507269,108.25018671496));
#46953=CARTESIAN_POINT('Ctrl Pts',(2.67844137132719,-8.7037887451894,108.18411989593));
#46954=CARTESIAN_POINT('Ctrl Pts',(2.73031217787741,-8.71444409330218,108.010482462731));
#46955=CARTESIAN_POINT('Ctrl Pts',(3.01369050100825,-8.73168869941104,107.869791362187));
#46956=CARTESIAN_POINT('Ctrl Pts',(3.32609103551689,-8.75145647339926,108.054013585571));
#46957=CARTESIAN_POINT('Ctrl Pts',(3.34216994997271,-8.77122424738748,108.416330284137));
#46958=CARTESIAN_POINT('Ctrl Pts',(3.04731620187133,-8.7909920213757,108.62750127831));
#46959=CARTESIAN_POINT('Ctrl Pts',(2.74253636262819,-8.80882482393743,108.508541612906));
#46960=CARTESIAN_POINT('Ctrl Pts',(2.6784894741245,-8.8200683685031,108.325221269276));
#46961=CARTESIAN_POINT('Ctrl Pts',(2.67787169029203,-8.82472265507269,108.249726345659));
#46962=CARTESIAN_POINT('Ctrl Pts',(2.67787688739042,-8.72437734492731,108.249727382091));
#46963=CARTESIAN_POINT('Ctrl Pts',(2.67761976356994,-8.72632421145764,108.218146907246));
#46964=CARTESIAN_POINT('Ctrl Pts',(2.69634964036998,-8.73486033598403,108.079979216136));
#46965=CARTESIAN_POINT('Ctrl Pts',(2.89355112400359,-8.7499857185065,107.884740242026));
#46966=CARTESIAN_POINT('Ctrl Pts',(3.2480100826438,-8.76975349249473,107.961491676198));
#46967=CARTESIAN_POINT('Ctrl Pts',(3.37710022867022,-8.78952126648294,108.300413009558));
#46968=CARTESIAN_POINT('Ctrl Pts',(3.16351627908797,-8.80928904047117,108.593523624325));
#46969=CARTESIAN_POINT('Ctrl Pts',(2.80134373476698,-8.82905681445938,108.574471481458));
#46970=CARTESIAN_POINT('Ctrl Pts',(2.67854928445123,-8.84241958261143,108.362277611636));
#46971=CARTESIAN_POINT('Ctrl Pts',(2.6771699054141,-8.84919309276741,108.253026234958));
#46972=CARTESIAN_POINT('Ctrl Pts',(2.67717687700499,-8.84937734492731,108.250054212538));
#46973=CARTESIAN_POINT('Origin',(3.,-7.51222265507269,108.25));
#46974=CARTESIAN_POINT('',(2.6772145464451,-8.5747226550727,108.250112544086));
#46975=CARTESIAN_POINT('',(2.67808628304073,-8.59937734492731,108.250189104615));
#46976=CARTESIAN_POINT('',(2.677725,-7.51222265507269,108.25));
#46977=CARTESIAN_POINT('Ctrl Pts',(2.6772145464451,-8.5747226550727,108.250112544086));
#46978=CARTESIAN_POINT('Ctrl Pts',(2.67766872176062,-8.58091986387963,108.150119216553));
#46979=CARTESIAN_POINT('Ctrl Pts',(2.78105395378419,-8.59370633068263,107.942995497513));
#46980=CARTESIAN_POINT('Ctrl Pts',(3.13308311396652,-8.61308205548171,107.893580411787));
#46981=CARTESIAN_POINT('Ctrl Pts',(3.37130152025498,-8.63284982946993,108.167046885883));
#46982=CARTESIAN_POINT('Ctrl Pts',(3.27211516521468,-8.65261760345815,108.515893540624));
#46983=CARTESIAN_POINT('Ctrl Pts',(2.92565550973071,-8.67238537744637,108.623120536626));
#46984=CARTESIAN_POINT('Ctrl Pts',(2.70412150102437,-8.68808706131789,108.438975741778));
#46985=CARTESIAN_POINT('Ctrl Pts',(2.67787154645913,-8.69719948719333,108.29118375902));
#46986=CARTESIAN_POINT('Ctrl Pts',(2.67808974459385,-8.69972265507269,108.25018671496));
#46987=CARTESIAN_POINT('Ctrl Pts',(2.67808628304073,-8.59937734492731,108.250189104615));
#46988=CARTESIAN_POINT('Ctrl Pts',(2.67844368879407,-8.60345533014786,108.183930786673));
#46989=CARTESIAN_POINT('Ctrl Pts',(2.73054658431704,-8.61412257336448,108.01009578156));
#46990=CARTESIAN_POINT('Ctrl Pts',(3.01437247462189,-8.63137907457718,107.869816510131));
#46991=CARTESIAN_POINT('Ctrl Pts',(3.32644207722428,-8.6511468485654,108.05459881215));
#46992=CARTESIAN_POINT('Ctrl Pts',(3.34187106527198,-8.67091462255362,108.41694378912));
#46993=CARTESIAN_POINT('Ctrl Pts',(3.04663898976117,-8.69068239654184,108.627585564647));
#46994=CARTESIAN_POINT('Ctrl Pts',(2.74227616279518,-8.70850330399974,108.508159103543));
#46995=CARTESIAN_POINT('Ctrl Pts',(2.67849001079218,-8.71973495346156,108.32503245546));
#46996=CARTESIAN_POINT('Ctrl Pts',(2.67787688739042,-8.72437734492731,108.249727382091));
#46997=CARTESIAN_POINT('Origin',(3.,-7.51222265507269,108.25));
#46998=CARTESIAN_POINT('',(2.67778257111066,-8.44972265507269,108.249714163392));
#46999=CARTESIAN_POINT('',(2.67721174697152,-8.47437734492731,108.250109332317));
#47000=CARTESIAN_POINT('',(2.677725,-7.51222265507269,108.25));
#47001=CARTESIAN_POINT('Ctrl Pts',(2.67778257111066,-8.44972265507269,108.249714163392));
#47002=CARTESIAN_POINT('Ctrl Pts',(2.67753611923224,-8.45146172457378,108.221525381468));
#47003=CARTESIAN_POINT('Ctrl Pts',(2.69379582962807,-8.45979005207093,108.086810217949));
#47004=CARTESIAN_POINT('Ctrl Pts',(2.8821598252778,-8.47470763756417,107.888254604305));
#47005=CARTESIAN_POINT('Ctrl Pts',(3.23884937624272,-8.49447541155238,107.9538631844));
#47006=CARTESIAN_POINT('Ctrl Pts',(3.37849452424005,-8.51424318554061,108.288573737252));
#47007=CARTESIAN_POINT('Ctrl Pts',(3.17419856871655,-8.53401095952883,108.58823201614));
#47008=CARTESIAN_POINT('Ctrl Pts',(2.81160693354902,-8.55377873351705,108.580536065503));
#47009=CARTESIAN_POINT('Ctrl Pts',(2.68021280133249,-8.56734929869834,108.369055249787));
#47010=CARTESIAN_POINT('Ctrl Pts',(2.67718581430621,-8.57433060588355,108.256438344007));
#47011=CARTESIAN_POINT('Ctrl Pts',(2.6772145464451,-8.5747226550727,108.250112544086));
#47012=CARTESIAN_POINT('Ctrl Pts',(2.67721174697152,-8.47437734492731,108.250109332317));
#47013=CARTESIAN_POINT('Ctrl Pts',(2.67765544676115,-8.48058644883809,108.14992636896));
#47014=CARTESIAN_POINT('Ctrl Pts',(2.78138880871222,-8.49338481074494,107.942633191673));
#47015=CARTESIAN_POINT('Ctrl Pts',(3.1337222307341,-8.51277243064786,107.893819681898));
#47016=CARTESIAN_POINT('Ctrl Pts',(3.37144973952803,-8.53254020463607,108.167713032621));
#47017=CARTESIAN_POINT('Ctrl Pts',(3.27163779891431,-8.5523079786243,108.51638123094));
#47018=CARTESIAN_POINT('Ctrl Pts',(2.92498634456088,-8.57207575261252,108.622986602298));
#47019=CARTESIAN_POINT('Ctrl Pts',(2.70395056442066,-8.58776554138019,108.438584522633));
#47020=CARTESIAN_POINT('Ctrl Pts',(2.67786618824155,-8.59686607215179,108.290991780691));
#47021=CARTESIAN_POINT('Ctrl Pts',(2.67808628304073,-8.59937734492731,108.250189104615));
#47022=CARTESIAN_POINT('Origin',(3.,-7.51222265507269,108.25));
#47023=CARTESIAN_POINT('',(2.67813962800902,-8.32472265507269,108.250144474503));
#47024=CARTESIAN_POINT('',(2.67778811510267,-8.34937734492731,108.249714634396));
#47025=CARTESIAN_POINT('',(2.677725,-7.51222265507269,108.25));
#47026=CARTESIAN_POINT('Ctrl Pts',(2.67813962800902,-8.32472265507269,108.250144474503));
#47027=CARTESIAN_POINT('Ctrl Pts',(2.67839617368377,-8.328592843264,108.187236279716));
#47028=CARTESIAN_POINT('Ctrl Pts',(2.72652582978869,-8.33905228945139,108.01686007521));
#47029=CARTESIAN_POINT('Ctrl Pts',(3.00245429834817,-8.35610099363484,107.869552875547));
#47030=CARTESIAN_POINT('Ctrl Pts',(3.32015990357356,-8.37586876762306,108.044467340237));
#47031=CARTESIAN_POINT('Ctrl Pts',(3.34693355738075,-8.39563654161128,108.406151032172));
#47032=CARTESIAN_POINT('Ctrl Pts',(3.05844581919422,-8.4154043155995,108.625938990135));
#47033=CARTESIAN_POINT('Ctrl Pts',(2.74689995323773,-8.43343302008664,108.514826151346));
#47034=CARTESIAN_POINT('Ctrl Pts',(2.67846991458055,-8.4448724665777,108.328331438717));
#47035=CARTESIAN_POINT('Ctrl Pts',(2.67778257111066,-8.44972265507269,108.249714163392));
#47036=CARTESIAN_POINT('Ctrl Pts',(2.67778811510267,-8.34937734492731,108.249714634396));
#47037=CARTESIAN_POINT('Ctrl Pts',(2.67754074084222,-8.35112830953224,108.221331794284));
#47038=CARTESIAN_POINT('Ctrl Pts',(2.69393854225206,-8.35946853213323,108.086419277493));
#47039=CARTESIAN_POINT('Ctrl Pts',(2.88280888503356,-8.37439801273031,107.888043791918));
#47040=CARTESIAN_POINT('Ctrl Pts',(3.23938019713941,-8.39416578671853,107.954292077865));
#47041=CARTESIAN_POINT('Ctrl Pts',(3.37842474494008,-8.41393356070675,108.289252597531));
#47042=CARTESIAN_POINT('Ctrl Pts',(3.17359159824674,-8.43370133469497,108.588543957285));
#47043=CARTESIAN_POINT('Ctrl Pts',(2.81101433099364,-8.45346910868319,108.580197624016));
#47044=CARTESIAN_POINT('Ctrl Pts',(2.68011458337086,-8.46702777876064,108.368667027259));
#47045=CARTESIAN_POINT('Ctrl Pts',(2.67718458133054,-8.47399719084201,108.256243061651));
#47046=CARTESIAN_POINT('Ctrl Pts',(2.67721174697152,-8.47437734492731,108.250109332317));
#47047=CARTESIAN_POINT('Origin',(3.,-7.51222265507269,108.25));
#47048=CARTESIAN_POINT('',(2.67726984584404,-8.19972265507269,108.250162467927));
#47049=CARTESIAN_POINT('',(2.67813696047442,-8.22437734492731,108.250147181483));
#47050=CARTESIAN_POINT('',(2.677725,-7.51222265507269,108.25));
#47051=CARTESIAN_POINT('Ctrl Pts',(2.67726984584404,-8.19972265507269,108.250162467927));
#47052=CARTESIAN_POINT('Ctrl Pts',(2.6778697318139,-8.20572396195423,108.153286050659));
#47053=CARTESIAN_POINT('Ctrl Pts',(2.77562443238243,-8.21831452683184,107.948991928386));
#47054=CARTESIAN_POINT('Ctrl Pts',(3.12249747634493,-8.23749434970551,107.889805043942));
#47055=CARTESIAN_POINT('Ctrl Pts',(3.36868932900526,-8.25726212369374,108.156115939767));
#47056=CARTESIAN_POINT('Ctrl Pts',(3.27985014011025,-8.27702989768196,108.507740057355));
#47057=CARTESIAN_POINT('Ctrl Pts',(2.93670881513792,-8.29679767167018,108.625153653859));
#47058=CARTESIAN_POINT('Ctrl Pts',(2.70700175452616,-8.31269525746709,108.445417818528));
#47059=CARTESIAN_POINT('Ctrl Pts',(2.67795938726534,-8.32200358526793,108.294341749793));
#47060=CARTESIAN_POINT('Ctrl Pts',(2.67813962800902,-8.32472265507269,108.250144474503));
#47061=CARTESIAN_POINT('Ctrl Pts',(2.67813696047442,-8.22437734492731,108.250147181483));
#47062=CARTESIAN_POINT('Ctrl Pts',(2.67839924484375,-8.22825942822246,108.187046934739));
#47063=CARTESIAN_POINT('Ctrl Pts',(2.72675174382006,-8.23873076951369,108.016472328973));
#47064=CARTESIAN_POINT('Ctrl Pts',(3.00313671720263,-8.25579136880099,107.869557869052));
#47065=CARTESIAN_POINT('Ctrl Pts',(3.32052807796508,-8.2755591427892,108.045041942749));
#47066=CARTESIAN_POINT('Ctrl Pts',(3.34665292419479,-8.29532691677743,108.406773097638));
#47067=CARTESIAN_POINT('Ctrl Pts',(3.05777139212753,-8.31509469076565,108.626043242523));
#47068=CARTESIAN_POINT('Ctrl Pts',(2.74663073970376,-8.33311150014894,108.51444542395));
#47069=CARTESIAN_POINT('Ctrl Pts',(2.67847166361423,-8.34453905153616,108.328142551985));
#47070=CARTESIAN_POINT('Ctrl Pts',(2.67778811510267,-8.34937734492731,108.249714634396));
#47071=CARTESIAN_POINT('Origin',(3.,-7.51222265507269,108.25));
#47072=CARTESIAN_POINT('',(2.67768910651924,-8.07472265507269,108.249711575117));
#47073=CARTESIAN_POINT('',(2.67726599767135,-8.09937734492731,108.250159613763));
#47074=CARTESIAN_POINT('',(2.677725,-7.51222265507269,108.25));
#47075=CARTESIAN_POINT('Ctrl Pts',(2.67768910651924,-8.07472265507269,108.249711575117));
#47076=CARTESIAN_POINT('Ctrl Pts',(2.67746272185417,-8.07626582264838,108.224716705907));
#47077=CARTESIAN_POINT('Ctrl Pts',(2.6915048408805,-8.08439824822013,108.093246364532));
#47078=CARTESIAN_POINT('Ctrl Pts',(2.87152636194084,-8.09911993178797,107.891893084811));
#47079=CARTESIAN_POINT('Ctrl Pts',(3.22999816400173,-8.11888770577619,107.946937494892));
#47080=CARTESIAN_POINT('Ctrl Pts',(3.37946873571844,-8.13865547976441,108.277377307303));
#47081=CARTESIAN_POINT('Ctrl Pts',(3.18411292856613,-8.15842325375263,108.582939135017));
#47082=CARTESIAN_POINT('Ctrl Pts',(2.8214521816118,-8.17819102774085,108.585956417675));
#47083=CARTESIAN_POINT('Ctrl Pts',(2.68188274081524,-8.19195749484754,108.375453327707));
#47084=CARTESIAN_POINT('Ctrl Pts',(2.67721107470776,-8.19913470395815,108.259653500236));
#47085=CARTESIAN_POINT('Ctrl Pts',(2.67726984584404,-8.19972265507269,108.250162467927));
#47086=CARTESIAN_POINT('Ctrl Pts',(2.67726599767135,-8.09937734492731,108.250159613763));
#47087=CARTESIAN_POINT('Ctrl Pts',(2.67785842523723,-8.10539054691269,108.153094218703));
#47088=CARTESIAN_POINT('Ctrl Pts',(2.77594951876704,-8.11799300689414,107.94862624596));
#47089=CARTESIAN_POINT('Ctrl Pts',(3.12314338152363,-8.13718472487166,107.890025332106));
#47090=CARTESIAN_POINT('Ctrl Pts',(3.36885715962375,-8.15695249885988,108.156777417877));
#47091=CARTESIAN_POINT('Ctrl Pts',(3.27938738699594,-8.1767202728481,108.508241634873));
#47092=CARTESIAN_POINT('Ctrl Pts',(2.93603598591862,-8.19648804683633,108.625039543106));
#47093=CARTESIAN_POINT('Ctrl Pts',(2.70682331429706,-8.2123737375294,108.445026745081));
#47094=CARTESIAN_POINT('Ctrl Pts',(2.67795405620495,-8.22167017022639,108.294150202185));
#47095=CARTESIAN_POINT('Ctrl Pts',(2.67813696047442,-8.22437734492731,108.250147181483));
#47096=CARTESIAN_POINT('Origin',(3.,-7.51222265507269,108.25));
#47097=CARTESIAN_POINT('',(2.67817606009431,-7.94972265507269,108.250097623709));
#47098=CARTESIAN_POINT('',(2.67769484037528,-7.97437734492731,108.249711449058));
#47099=CARTESIAN_POINT('',(2.677725,-7.51222265507269,108.25));
#47100=CARTESIAN_POINT('Ctrl Pts',(2.67817606009431,-7.94972265507269,108.250097623709));
#47101=CARTESIAN_POINT('Ctrl Pts',(2.67833968674077,-7.9533969413386,108.190356954968));
#47102=CARTESIAN_POINT('Ctrl Pts',(2.7228778240257,-7.96366048560059,108.023254014987));
#47103=CARTESIAN_POINT('Ctrl Pts',(2.99121613241808,-7.98051328785865,107.869646268722));
#47104=CARTESIAN_POINT('Ctrl Pts',(3.31394930971311,-8.00028106184687,108.035100497677));
#47105=CARTESIAN_POINT('Ctrl Pts',(3.35139445931568,-8.02004883583509,108.395835495957));
#47106=CARTESIAN_POINT('Ctrl Pts',(3.0695244178543,-8.03981660982331,108.624048658391));
#47107=CARTESIAN_POINT('Ctrl Pts',(2.75141308756519,-8.05804121623585,108.521079574909));
#47108=CARTESIAN_POINT('Ctrl Pts',(2.67842937446406,-8.0696765646523,108.331443703284));
#47109=CARTESIAN_POINT('Ctrl Pts',(2.67768910651924,-8.07472265507269,108.249711575117));
#47110=CARTESIAN_POINT('Ctrl Pts',(2.67769484037528,-7.97437734492731,108.249711449058));
#47111=CARTESIAN_POINT('Ctrl Pts',(2.67746698787036,-7.97593240760684,108.224522765322));
#47112=CARTESIAN_POINT('Ctrl Pts',(2.69164072765528,-7.98407672828244,108.09285569702));
#47113=CARTESIAN_POINT('Ctrl Pts',(2.87216892550497,-7.99881030695412,107.891663181036));
#47114=CARTESIAN_POINT('Ctrl Pts',(3.23054141520414,-8.01857808094234,107.94735052791));
#47115=CARTESIAN_POINT('Ctrl Pts',(3.37941904127915,-8.03834585493056,108.278057929909));
#47116=CARTESIAN_POINT('Ctrl Pts',(3.18351543540106,-8.05811362891878,108.583268869327));
#47117=CARTESIAN_POINT('Ctrl Pts',(2.82084984167802,-8.07788140290699,108.585635627028));
#47118=CARTESIAN_POINT('Ctrl Pts',(2.68177847505825,-8.09163597490984,108.375064617705));
#47119=CARTESIAN_POINT('Ctrl Pts',(2.67720924397156,-8.09880128891661,108.259458337536));
#47120=CARTESIAN_POINT('Ctrl Pts',(2.67726599767135,-8.09937734492731,108.250159613763));
#47121=CARTESIAN_POINT('Origin',(3.,-7.51222265507269,108.25));
#47122=CARTESIAN_POINT('',(2.67736158403691,-7.82472265507269,108.25018840343));
#47123=CARTESIAN_POINT('',(2.6781760831613,-7.84937734492731,108.250099030543));
#47124=CARTESIAN_POINT('',(2.677725,-7.51222265507269,108.25));
#47125=CARTESIAN_POINT('Ctrl Pts',(2.67736158403691,-7.82472265507269,108.25018840343));
#47126=CARTESIAN_POINT('Ctrl Pts',(2.67807187286672,-7.83052806002883,108.156415124274));
#47127=CARTESIAN_POINT('Ctrl Pts',(2.77031473193814,-7.84292272298104,107.955065044056));
#47128=CARTESIAN_POINT('Ctrl Pts',(3.1118235245366,-7.86190664392932,107.886332436713));
#47129=CARTESIAN_POINT('Ctrl Pts',(3.3657465801897,-7.88167441791754,108.145272177939));
#47130=CARTESIAN_POINT('Ctrl Pts',(3.28734488563378,-7.90144219190576,108.499359232776));
#47131=CARTESIAN_POINT('Ctrl Pts',(2.94781550033985,-7.92120996589399,108.626860515219));
#47132=CARTESIAN_POINT('Ctrl Pts',(2.71000718921594,-7.93730345361629,108.451856374517));
#47133=CARTESIAN_POINT('Ctrl Pts',(2.67804624793102,-7.94680768334253,108.297492504759));
#47134=CARTESIAN_POINT('Ctrl Pts',(2.67817606009431,-7.94972265507269,108.250097623709));
#47135=CARTESIAN_POINT('Ctrl Pts',(2.6781760831613,-7.84937734492731,108.250099030543));
#47136=CARTESIAN_POINT('Ctrl Pts',(2.67834452920302,-7.85306352629706,108.190166386294));
#47137=CARTESIAN_POINT('Ctrl Pts',(2.72309291261354,-7.86333896566289,108.022867558002));
#47138=CARTESIAN_POINT('Ctrl Pts',(2.99189987276353,-7.88020366302479,107.869629820223));
#47139=CARTESIAN_POINT('Ctrl Pts',(3.31433362603907,-7.89997143701301,108.035664564453));
#47140=CARTESIAN_POINT('Ctrl Pts',(3.35113263206487,-7.91973921100123,108.396465308122));
#47141=CARTESIAN_POINT('Ctrl Pts',(3.06885322266343,-7.93950698498945,108.624172910368));
#47142=CARTESIAN_POINT('Ctrl Pts',(2.75113478560957,-7.95771969629815,108.520700790562));
#47143=CARTESIAN_POINT('Ctrl Pts',(2.67843246595669,-7.96934314961076,108.33125462758));
#47144=CARTESIAN_POINT('Ctrl Pts',(2.67769484037528,-7.97437734492731,108.249711449058));
#47145=CARTESIAN_POINT('Origin',(3.78136533198136,-11.25,107.59435663812));
#47146=CARTESIAN_POINT('',(3.78136533198136,-11.16,107.59435663812));
#47147=CARTESIAN_POINT('',(3.88624986816126,-11.,107.598416412742));
#47148=CARTESIAN_POINT('Ctrl Pts',(3.78136533198136,-11.16,107.59435663812));
#47149=CARTESIAN_POINT('Ctrl Pts',(3.83182864655857,-11.0851968149525,107.59630992591));
#47150=CARTESIAN_POINT('Ctrl Pts',(3.88624986816125,-11.,107.598416412742));
#47151=CARTESIAN_POINT('',(3.78136533198136,-9.9,107.59435663812));
#47152=CARTESIAN_POINT('',(3.78136533198136,-11.25,107.59435663812));
#47153=CARTESIAN_POINT('',(3.88624986816126,-9.9,107.598416412742));
#47154=CARTESIAN_POINT('',(3.78136533198136,-9.9,107.59435663812));
#47155=CARTESIAN_POINT('',(3.88624986816126,-10.4,107.598416412742));
#47156=CARTESIAN_POINT('Origin',(3.8715244580726,-9.9,107.508451031791));
#47157=CARTESIAN_POINT('',(3.79558024303105,-9.9,107.490360561254));
#47158=CARTESIAN_POINT('Origin',(3.,-9.9,108.25));
#47159=CARTESIAN_POINT('',(3.80580370973244,-9.9,107.415565831607));
#47160=CARTESIAN_POINT('Origin',(3.80580370973244,-11.25,107.415565831607));
#47161=CARTESIAN_POINT('',(3.79558024303105,-11.,107.490360561254));
#47162=CARTESIAN_POINT('Ctrl Pts',(3.79558024303106,-11.,107.490360561254));
#47163=CARTESIAN_POINT('Ctrl Pts',(3.78820458163732,-11.085196814953,107.544320789817));
#47164=CARTESIAN_POINT('Ctrl Pts',(3.78136533198136,-11.16,107.59435663812));
#47165=CARTESIAN_POINT('',(3.79558024303105,-10.4,107.490360561254));
#47166=CARTESIAN_POINT('Origin',(3.17712114122027,-11.25,107.245496091928));
#47167=CARTESIAN_POINT('',(3.17712114122027,-11.16,107.245496091928));
#47168=CARTESIAN_POINT('',(3.26007693015524,-11.,107.181187579413));
#47169=CARTESIAN_POINT('Ctrl Pts',(3.17712114122027,-11.16,107.245496091928));
#47170=CARTESIAN_POINT('Ctrl Pts',(3.21703383212295,-11.0851968149527,107.214555203831));
#47171=CARTESIAN_POINT('Ctrl Pts',(3.26007693015524,-11.,107.181187579413));
#47172=CARTESIAN_POINT('',(3.17712114122027,-9.9,107.245496091928));
#47173=CARTESIAN_POINT('',(3.17712114122027,-11.25,107.245496091928));
#47174=CARTESIAN_POINT('',(3.26007693015524,-9.9,107.181187579413));
#47175=CARTESIAN_POINT('',(3.17712114122027,-9.9,107.245496091928));
#47176=CARTESIAN_POINT('',(3.26007693015524,-10.4,107.181187579413));
#47177=CARTESIAN_POINT('Origin',(3.20032842114545,-9.9,107.169160896813));
#47178=CARTESIAN_POINT('',(3.12116300517389,-9.9,107.156693306443));
#47179=CARTESIAN_POINT('Origin',(3.,-9.9,108.25));
#47180=CARTESIAN_POINT('',(3.08091750954319,-9.9,107.092825701699));
#47181=CARTESIAN_POINT('Origin',(3.08091750954319,-11.25,107.092825701699));
#47182=CARTESIAN_POINT('',(3.12116300517389,-11.,107.156693306443));
#47183=CARTESIAN_POINT('Ctrl Pts',(3.12116300517389,-11.,107.156693306443));
#47184=CARTESIAN_POINT('Ctrl Pts',(3.15019788708483,-11.0851968149529,107.20277022344));
#47185=CARTESIAN_POINT('Ctrl Pts',(3.17712114122027,-11.16,107.245496091928));
#47186=CARTESIAN_POINT('',(3.12116300517389,-10.4,107.156693306443));
#47187=CARTESIAN_POINT('Origin',(2.49,-11.25,107.36665408814));
#47188=CARTESIAN_POINT('',(2.49,-11.16,107.36665408814));
#47189=CARTESIAN_POINT('',(2.51221110609647,-11.,107.264067956204));
#47190=CARTESIAN_POINT('Ctrl Pts',(2.49,-11.16,107.36665408814));
#47191=CARTESIAN_POINT('Ctrl Pts',(2.50068647557472,-11.0851968149526,107.317296609567));
#47192=CARTESIAN_POINT('Ctrl Pts',(2.51221110609647,-11.,107.264067956204));
#47193=CARTESIAN_POINT('',(2.49,-9.9,107.36665408814));
#47194=CARTESIAN_POINT('',(2.49,-11.25,107.36665408814));
#47195=CARTESIAN_POINT('',(2.51221110609646,-9.9,107.264067956204));
#47196=CARTESIAN_POINT('',(2.49,-9.9,107.36665408814));
#47197=CARTESIAN_POINT('',(2.51221110609647,-10.4,107.264067956204));
#47198=CARTESIAN_POINT('Origin',(2.4231773006864,-9.9,107.278470678637));
#47199=CARTESIAN_POINT('',(2.39005225061905,-9.9,107.334596404297));
#47200=CARTESIAN_POINT('Origin',(3.,-9.9,108.25));
#47201=CARTESIAN_POINT('',(2.31816910734073,-9.9,107.311540286525));
#47202=CARTESIAN_POINT('Origin',(2.31816910734073,-11.25,107.311540286525));
#47203=CARTESIAN_POINT('',(2.39005225061905,-11.,107.334596404297));
#47204=CARTESIAN_POINT('Ctrl Pts',(2.39005225061905,-11.,107.334596404297));
#47205=CARTESIAN_POINT('Ctrl Pts',(2.44191193190111,-11.0851968149519,107.351230108178));
#47206=CARTESIAN_POINT('Ctrl Pts',(2.49,-11.16,107.36665408814));
#47207=CARTESIAN_POINT('',(2.39005225061905,-10.4,107.334596404297));
#47208=CARTESIAN_POINT('Origin',(2.04151352679837,-11.25,107.901139453808));
#47209=CARTESIAN_POINT('',(2.04151352679837,-11.16,107.901139453808));
#47210=CARTESIAN_POINT('',(1.99258712666485,-11.,107.808276893701));
#47211=CARTESIAN_POINT('Ctrl Pts',(2.04151352679837,-11.16,107.901139453808));
#47212=CARTESIAN_POINT('Ctrl Pts',(2.01797346635675,-11.0851968149526,107.85646029753));
#47213=CARTESIAN_POINT('Ctrl Pts',(1.99258712666485,-11.,107.808276893701));
#47214=CARTESIAN_POINT('',(2.04151352679837,-9.9,107.901139453808));
#47215=CARTESIAN_POINT('',(2.04151352679837,-11.25,107.901139453808));
#47216=CARTESIAN_POINT('',(1.99258712666485,-9.9,107.808276893701));
#47217=CARTESIAN_POINT('',(2.04151352679837,-9.9,107.901139453808));
#47218=CARTESIAN_POINT('',(1.99258712666485,-10.4,107.808276893701));
#47219=CARTESIAN_POINT('Origin',(1.95798524215911,-9.9,107.855430035415));
#47220=CARTESIAN_POINT('',(1.94434282681371,-9.9,107.940827018159));
#47221=CARTESIAN_POINT('Origin',(3.,-9.9,108.25));
#47222=CARTESIAN_POINT('',(1.87445695751984,-9.9,107.969370601104));
#47223=CARTESIAN_POINT('Origin',(1.87445695751984,-11.25,107.969370601104));
#47224=CARTESIAN_POINT('',(1.94434282681371,-11.,107.940827018159));
#47225=CARTESIAN_POINT('Ctrl Pts',(1.94434282681371,-11.,107.940827018159));
#47226=CARTESIAN_POINT('Ctrl Pts',(1.99476158623952,-11.0851968149524,107.920234414015));
#47227=CARTESIAN_POINT('Ctrl Pts',(2.04151352679837,-11.16,107.901139453808));
#47228=CARTESIAN_POINT('',(1.94434282681371,-10.4,107.940827018159));
#47229=CARTESIAN_POINT('Origin',(4.02,-11.25,108.25));
#47230=CARTESIAN_POINT('',(4.02,-11.16,108.25));
#47231=CARTESIAN_POINT('',(4.09773664328448,-11.,108.320528448094));
#47232=CARTESIAN_POINT('Ctrl Pts',(4.02,-11.16,108.25));
#47233=CARTESIAN_POINT('Ctrl Pts',(4.05740159252348,-11.0851968149531,108.283933498611));
#47234=CARTESIAN_POINT('Ctrl Pts',(4.09773664328448,-11.,108.320528448094));
#47235=CARTESIAN_POINT('',(4.02,-9.9,108.25));
#47236=CARTESIAN_POINT('',(4.02,-11.25,108.25));
#47237=CARTESIAN_POINT('',(4.09773664328448,-9.9,108.320528448094));
#47238=CARTESIAN_POINT('',(4.02,-9.9,108.25));
#47239=CARTESIAN_POINT('',(4.09773664328448,-10.4,108.320528448094));
#47240=CARTESIAN_POINT('Origin',(4.0868226993136,-9.9,108.25));
#47241=CARTESIAN_POINT('',(4.09773664328448,-9.9,108.179471551906));
#47242=CARTESIAN_POINT('Origin',(3.,-9.9,108.25));
#47243=CARTESIAN_POINT('',(4.1536453986272,-9.9,108.12874698261));
#47244=CARTESIAN_POINT('Origin',(4.1536453986272,-11.25,108.12874698261));
#47245=CARTESIAN_POINT('',(4.09773664328448,-11.,108.179471551906));
#47246=CARTESIAN_POINT('Ctrl Pts',(4.09773664328448,-11.,108.179471551906));
#47247=CARTESIAN_POINT('Ctrl Pts',(4.05740159252348,-11.0851968149531,108.216066501389));
#47248=CARTESIAN_POINT('Ctrl Pts',(4.02,-11.16,108.25));
#47249=CARTESIAN_POINT('',(4.09773664328448,-10.4,108.179471551906));
#47250=CARTESIAN_POINT('Origin',(2.21863466801864,-11.25,108.90564336188));
#47251=CARTESIAN_POINT('',(2.21863466801864,-11.16,108.90564336188));
#47252=CARTESIAN_POINT('',(2.11375013183874,-11.,108.901583587258));
#47253=CARTESIAN_POINT('Ctrl Pts',(2.21863466801864,-11.16,108.90564336188));
#47254=CARTESIAN_POINT('Ctrl Pts',(2.16817135344143,-11.0851968149525,108.90369007409));
#47255=CARTESIAN_POINT('Ctrl Pts',(2.11375013183875,-11.,108.901583587258));
#47256=CARTESIAN_POINT('',(2.21863466801864,-9.9,108.90564336188));
#47257=CARTESIAN_POINT('',(2.21863466801864,-11.25,108.90564336188));
#47258=CARTESIAN_POINT('',(2.11375013183874,-9.9,108.901583587258));
#47259=CARTESIAN_POINT('',(2.21863466801864,-9.9,108.90564336188));
#47260=CARTESIAN_POINT('',(2.11375013183874,-10.4,108.901583587258));
#47261=CARTESIAN_POINT('Origin',(2.1284755419274,-9.9,108.991548968209));
#47262=CARTESIAN_POINT('',(2.20441975696894,-9.9,109.009639438746));
#47263=CARTESIAN_POINT('Origin',(3.,-9.9,108.25));
#47264=CARTESIAN_POINT('',(2.19419629026756,-9.9,109.084434168393));
#47265=CARTESIAN_POINT('Origin',(2.19419629026756,-11.25,109.084434168393));
#47266=CARTESIAN_POINT('',(2.20441975696894,-11.,109.009639438746));
#47267=CARTESIAN_POINT('Ctrl Pts',(2.20441975696894,-11.,109.009639438746));
#47268=CARTESIAN_POINT('Ctrl Pts',(2.21179541836267,-11.0851968149528,108.955679210184));
#47269=CARTESIAN_POINT('Ctrl Pts',(2.21863466801864,-11.16,108.90564336188));
#47270=CARTESIAN_POINT('',(2.20441975696894,-10.4,109.009639438746));
#47271=CARTESIAN_POINT('Origin',(2.82287885877973,-11.25,109.254503908072));
#47272=CARTESIAN_POINT('',(2.82287885877973,-11.16,109.254503908072));
#47273=CARTESIAN_POINT('',(2.73992306984476,-11.,109.318812420587));
#47274=CARTESIAN_POINT('Ctrl Pts',(2.82287885877973,-11.16,109.254503908072));
#47275=CARTESIAN_POINT('Ctrl Pts',(2.78296616787725,-11.0851968149531,109.285444796169));
#47276=CARTESIAN_POINT('Ctrl Pts',(2.73992306984476,-11.,109.318812420587));
#47277=CARTESIAN_POINT('',(2.82287885877973,-9.9,109.254503908072));
#47278=CARTESIAN_POINT('',(2.82287885877973,-11.25,109.254503908072));
#47279=CARTESIAN_POINT('',(2.73992306984476,-9.9,109.318812420587));
#47280=CARTESIAN_POINT('',(2.82287885877973,-9.9,109.254503908072));
#47281=CARTESIAN_POINT('',(2.73992306984476,-10.4,109.318812420587));
#47282=CARTESIAN_POINT('Origin',(2.79967157885455,-9.9,109.330839103187));
#47283=CARTESIAN_POINT('',(2.87883699482611,-9.9,109.343306693557));
#47284=CARTESIAN_POINT('Origin',(3.,-9.9,108.25));
#47285=CARTESIAN_POINT('',(2.91908249045681,-9.9,109.407174298301));
#47286=CARTESIAN_POINT('Origin',(2.91908249045681,-11.25,109.407174298301));
#47287=CARTESIAN_POINT('',(2.87883699482611,-11.,109.343306693557));
#47288=CARTESIAN_POINT('Ctrl Pts',(2.87883699482611,-11.,109.343306693557));
#47289=CARTESIAN_POINT('Ctrl Pts',(2.84980211291528,-11.0851968149526,109.29722977656));
#47290=CARTESIAN_POINT('Ctrl Pts',(2.82287885877973,-11.16,109.254503908072));
#47291=CARTESIAN_POINT('',(2.87883699482611,-10.4,109.343306693557));
#47292=CARTESIAN_POINT('Origin',(3.51,-11.25,109.13334591186));
#47293=CARTESIAN_POINT('',(3.51,-11.16,109.13334591186));
#47294=CARTESIAN_POINT('',(3.48778889390354,-11.,109.235932043796));
#47295=CARTESIAN_POINT('Ctrl Pts',(3.51,-11.16,109.13334591186));
#47296=CARTESIAN_POINT('Ctrl Pts',(3.49931352442526,-11.0851968149525,109.182703390433));
#47297=CARTESIAN_POINT('Ctrl Pts',(3.48778889390353,-11.,109.235932043796));
#47298=CARTESIAN_POINT('',(3.51,-9.9,109.13334591186));
#47299=CARTESIAN_POINT('',(3.51,-11.25,109.13334591186));
#47300=CARTESIAN_POINT('',(3.48778889390354,-9.9,109.235932043796));
#47301=CARTESIAN_POINT('',(3.51,-9.9,109.13334591186));
#47302=CARTESIAN_POINT('',(3.48778889390354,-10.4,109.235932043796));
#47303=CARTESIAN_POINT('Origin',(3.5768226993136,-9.9,109.221529321363));
#47304=CARTESIAN_POINT('',(3.60994774938095,-9.9,109.165403595703));
#47305=CARTESIAN_POINT('Origin',(3.,-9.9,108.25));
#47306=CARTESIAN_POINT('',(3.68183089265927,-9.9,109.188459713475));
#47307=CARTESIAN_POINT('Origin',(3.68183089265927,-11.25,109.188459713475));
#47308=CARTESIAN_POINT('',(3.60994774938095,-11.,109.165403595703));
#47309=CARTESIAN_POINT('Ctrl Pts',(3.60994774938095,-11.,109.165403595703));
#47310=CARTESIAN_POINT('Ctrl Pts',(3.55808806809889,-11.0851968149519,109.148769891822));
#47311=CARTESIAN_POINT('Ctrl Pts',(3.51,-11.16,109.13334591186));
#47312=CARTESIAN_POINT('',(3.60994774938095,-10.4,109.165403595703));
#47313=CARTESIAN_POINT('Origin',(3.95848647320163,-11.25,108.598860546192));
#47314=CARTESIAN_POINT('',(3.95848647320163,-11.16,108.598860546192));
#47315=CARTESIAN_POINT('',(4.00741287333515,-11.,108.691723106299));
#47316=CARTESIAN_POINT('Ctrl Pts',(3.95848647320162,-11.16,108.598860546192));
#47317=CARTESIAN_POINT('Ctrl Pts',(3.98202653364333,-11.0851968149524,108.64353970247));
#47318=CARTESIAN_POINT('Ctrl Pts',(4.00741287333515,-11.,108.691723106299));
#47319=CARTESIAN_POINT('',(3.95848647320163,-9.9,108.598860546192));
#47320=CARTESIAN_POINT('',(3.95848647320163,-11.25,108.598860546192));
#47321=CARTESIAN_POINT('',(4.00741287333515,-9.9,108.691723106299));
#47322=CARTESIAN_POINT('',(3.95848647320163,-9.9,108.598860546192));
#47323=CARTESIAN_POINT('',(4.00741287333515,-10.4,108.691723106299));
#47324=CARTESIAN_POINT('Origin',(4.04201475784089,-9.9,108.644569964585));
#47325=CARTESIAN_POINT('',(4.05565717318629,-9.9,108.559172981841));
#47326=CARTESIAN_POINT('Origin',(3.,-9.9,108.25));
#47327=CARTESIAN_POINT('',(4.12554304248016,-9.9,108.530629398896));
#47328=CARTESIAN_POINT('Origin',(4.12554304248016,-11.25,108.530629398896));
#47329=CARTESIAN_POINT('',(4.05565717318629,-11.,108.559172981841));
#47330=CARTESIAN_POINT('Ctrl Pts',(4.05565717318629,-11.,108.559172981841));
#47331=CARTESIAN_POINT('Ctrl Pts',(4.00523841376048,-11.0851968149523,108.579765585985));
#47332=CARTESIAN_POINT('Ctrl Pts',(3.95848647320163,-11.16,108.598860546192));
#47333=CARTESIAN_POINT('',(4.05565717318629,-10.4,108.559172981841));
#47334=CARTESIAN_POINT('Origin',(3.78136533198136,-11.25,108.90564336188));
#47335=CARTESIAN_POINT('',(3.78136533198136,-11.16,108.90564336188));
#47336=CARTESIAN_POINT('',(3.79558024303105,-11.,109.009639438746));
#47337=CARTESIAN_POINT('Ctrl Pts',(3.78136533198136,-11.16,108.90564336188));
#47338=CARTESIAN_POINT('Ctrl Pts',(3.78820458163732,-11.085196814953,108.955679210183));
#47339=CARTESIAN_POINT('Ctrl Pts',(3.79558024303106,-11.,109.009639438746));
#47340=CARTESIAN_POINT('',(3.78136533198136,-9.9,108.90564336188));
#47341=CARTESIAN_POINT('',(3.78136533198136,-11.25,108.90564336188));
#47342=CARTESIAN_POINT('',(3.79558024303105,-9.9,109.009639438746));
#47343=CARTESIAN_POINT('',(3.78136533198136,-9.9,108.90564336188));
#47344=CARTESIAN_POINT('',(3.79558024303105,-10.4,109.009639438746));
#47345=CARTESIAN_POINT('Origin',(3.8715244580726,-9.9,108.991548968209));
#47346=CARTESIAN_POINT('',(3.88624986816126,-9.9,108.901583587258));
#47347=CARTESIAN_POINT('Origin',(3.,-9.9,108.25));
#47348=CARTESIAN_POINT('',(3.96168358416385,-9.9,108.898663768026));
#47349=CARTESIAN_POINT('Origin',(3.96168358416385,-11.25,108.898663768026));
#47350=CARTESIAN_POINT('',(3.88624986816126,-11.,108.901583587258));
#47351=CARTESIAN_POINT('Ctrl Pts',(3.88624986816126,-11.,108.901583587258));
#47352=CARTESIAN_POINT('Ctrl Pts',(3.83182864655864,-11.0851968149524,108.90369007409));
#47353=CARTESIAN_POINT('Ctrl Pts',(3.78136533198136,-11.16,108.90564336188));
#47354=CARTESIAN_POINT('',(3.88624986816126,-10.4,108.901583587258));
#47355=CARTESIAN_POINT('Origin',(3.17712114122027,-11.25,109.254503908072));
#47356=CARTESIAN_POINT('',(3.17712114122027,-11.16,109.254503908072));
#47357=CARTESIAN_POINT('',(3.12116300517389,-11.,109.343306693557));
#47358=CARTESIAN_POINT('Ctrl Pts',(3.17712114122027,-11.16,109.254503908072));
#47359=CARTESIAN_POINT('Ctrl Pts',(3.15019788708492,-11.0851968149532,109.29722977656));
#47360=CARTESIAN_POINT('Ctrl Pts',(3.12116300517389,-11.,109.343306693557));
#47361=CARTESIAN_POINT('',(3.17712114122027,-9.9,109.254503908072));
#47362=CARTESIAN_POINT('',(3.17712114122027,-11.25,109.254503908072));
#47363=CARTESIAN_POINT('',(3.12116300517389,-9.9,109.343306693557));
#47364=CARTESIAN_POINT('',(3.17712114122027,-9.9,109.254503908072));
#47365=CARTESIAN_POINT('',(3.12116300517389,-10.4,109.343306693557));
#47366=CARTESIAN_POINT('Origin',(3.20032842114545,-9.9,109.330839103187));
#47367=CARTESIAN_POINT('',(3.26007693015523,-9.9,109.318812420587));
#47368=CARTESIAN_POINT('Origin',(3.,-9.9,108.25));
#47369=CARTESIAN_POINT('',(3.31973933274772,-9.9,109.365063567288));
#47370=CARTESIAN_POINT('Origin',(3.31973933274772,-11.25,109.365063567288));
#47371=CARTESIAN_POINT('',(3.26007693015523,-11.,109.318812420587));
#47372=CARTESIAN_POINT('Ctrl Pts',(3.26007693015523,-11.,109.318812420587));
#47373=CARTESIAN_POINT('Ctrl Pts',(3.2170338321225,-11.0851968149535,109.285444796169));
#47374=CARTESIAN_POINT('Ctrl Pts',(3.17712114122027,-11.16,109.254503908072));
#47375=CARTESIAN_POINT('',(3.26007693015523,-10.4,109.318812420587));
#47376=CARTESIAN_POINT('Origin',(2.49,-11.25,109.13334591186));
#47377=CARTESIAN_POINT('',(2.49,-11.16,109.13334591186));
#47378=CARTESIAN_POINT('',(2.39005225061905,-11.,109.165403595703));
#47379=CARTESIAN_POINT('Ctrl Pts',(2.49,-11.16,109.13334591186));
#47380=CARTESIAN_POINT('Ctrl Pts',(2.4419119319011,-11.0851968149518,109.148769891822));
#47381=CARTESIAN_POINT('Ctrl Pts',(2.39005225061905,-11.,109.165403595703));
#47382=CARTESIAN_POINT('',(2.49,-9.9,109.13334591186));
#47383=CARTESIAN_POINT('',(2.49,-11.25,109.13334591186));
#47384=CARTESIAN_POINT('',(2.39005225061905,-9.9,109.165403595703));
#47385=CARTESIAN_POINT('',(2.49,-9.9,109.13334591186));
#47386=CARTESIAN_POINT('',(2.39005225061905,-10.4,109.165403595703));
#47387=CARTESIAN_POINT('Origin',(2.4231773006864,-9.9,109.221529321363));
#47388=CARTESIAN_POINT('',(2.51221110609646,-9.9,109.235932043796));
#47389=CARTESIAN_POINT('Origin',(3.,-9.9,108.25));
#47390=CARTESIAN_POINT('',(2.52818549403207,-9.9,109.309712730865));
#47391=CARTESIAN_POINT('Origin',(2.52818549403207,-11.25,109.309712730865));
#47392=CARTESIAN_POINT('',(2.51221110609646,-11.,109.235932043796));
#47393=CARTESIAN_POINT('Ctrl Pts',(2.51221110609647,-11.,109.235932043796));
#47394=CARTESIAN_POINT('Ctrl Pts',(2.5006864755747,-11.0851968149528,109.182703390433));
#47395=CARTESIAN_POINT('Ctrl Pts',(2.49,-11.16,109.13334591186));
#47396=CARTESIAN_POINT('',(2.51221110609646,-10.4,109.235932043796));
#47397=CARTESIAN_POINT('Origin',(2.04151352679837,-11.25,108.598860546192));
#47398=CARTESIAN_POINT('',(2.04151352679837,-11.16,108.598860546192));
#47399=CARTESIAN_POINT('',(1.94434282681371,-11.,108.559172981841));
#47400=CARTESIAN_POINT('Ctrl Pts',(2.04151352679837,-11.16,108.598860546192));
#47401=CARTESIAN_POINT('Ctrl Pts',(1.99476158623951,-11.0851968149523,108.579765585985));
#47402=CARTESIAN_POINT('Ctrl Pts',(1.94434282681371,-11.,108.559172981841));
#47403=CARTESIAN_POINT('',(2.04151352679837,-9.9,108.598860546192));
#47404=CARTESIAN_POINT('',(2.04151352679837,-11.25,108.598860546192));
#47405=CARTESIAN_POINT('',(1.94434282681371,-9.9,108.559172981841));
#47406=CARTESIAN_POINT('',(2.04151352679837,-9.9,108.598860546192));
#47407=CARTESIAN_POINT('',(1.94434282681371,-10.4,108.559172981841));
#47408=CARTESIAN_POINT('Origin',(1.95798524215911,-9.9,108.644569964585));
#47409=CARTESIAN_POINT('',(1.99258712666485,-9.9,108.691723106299));
#47410=CARTESIAN_POINT('Origin',(3.,-9.9,108.25));
#47411=CARTESIAN_POINT('',(1.95739890629297,-9.9,108.758510530275));
#47412=CARTESIAN_POINT('Origin',(1.95739890629297,-11.25,108.758510530275));
#47413=CARTESIAN_POINT('',(1.99258712666485,-11.,108.691723106299));
#47414=CARTESIAN_POINT('Ctrl Pts',(1.99258712666485,-11.,108.691723106299));
#47415=CARTESIAN_POINT('Ctrl Pts',(2.01797346635666,-11.0851968149523,108.64353970247));
#47416=CARTESIAN_POINT('Ctrl Pts',(2.04151352679837,-11.16,108.598860546192));
#47417=CARTESIAN_POINT('',(1.99258712666485,-10.4,108.691723106299));
#47418=CARTESIAN_POINT('Origin',(1.98,-11.25,108.25));
#47419=CARTESIAN_POINT('',(1.98,-11.16,108.25));
#47420=CARTESIAN_POINT('',(1.90226335671552,-11.,108.179471551906));
#47421=CARTESIAN_POINT('Ctrl Pts',(1.98,-11.16,108.25));
#47422=CARTESIAN_POINT('Ctrl Pts',(1.94259840747653,-11.0851968149531,108.216066501389));
#47423=CARTESIAN_POINT('Ctrl Pts',(1.90226335671552,-11.,108.179471551906));
#47424=CARTESIAN_POINT('',(1.98,-9.9,108.25));
#47425=CARTESIAN_POINT('',(1.98,-11.25,108.25));
#47426=CARTESIAN_POINT('',(1.90226335671552,-9.9,108.179471551906));
#47427=CARTESIAN_POINT('',(1.98,-9.9,108.25));
#47428=CARTESIAN_POINT('',(1.90226335671552,-10.4,108.179471551906));
#47429=CARTESIAN_POINT('Origin',(1.9131773006864,-9.9,108.25));
#47430=CARTESIAN_POINT('',(1.9,-9.9,108.25));
#47431=CARTESIAN_POINT('Origin',(3.,-9.9,108.25));
#47432=CARTESIAN_POINT('',(1.90226335671552,-9.9,108.320528448094));
#47433=CARTESIAN_POINT('',(1.8463546013728,-9.9,108.37125301739));
#47434=CARTESIAN_POINT('Origin',(3.,-9.9,108.25));
#47435=CARTESIAN_POINT('Origin',(1.8463546013728,-11.25,108.37125301739));
#47436=CARTESIAN_POINT('',(1.90226335671552,-11.,108.320528448094));
#47437=CARTESIAN_POINT('Ctrl Pts',(1.90226335671552,-11.,108.320528448094));
#47438=CARTESIAN_POINT('Ctrl Pts',(1.94259840747628,-11.0851968149526,108.283933498611));
#47439=CARTESIAN_POINT('Ctrl Pts',(1.98,-11.16,108.25));
#47440=CARTESIAN_POINT('',(1.90226335671552,-10.4,108.320528448094));
#47441=CARTESIAN_POINT('Origin',(2.21863466801864,-11.25,107.59435663812));
#47442=CARTESIAN_POINT('',(2.21863466801864,-11.16,107.59435663812));
#47443=CARTESIAN_POINT('',(2.20441975696895,-11.,107.490360561254));
#47444=CARTESIAN_POINT('Ctrl Pts',(2.21863466801864,-11.16,107.59435663812));
#47445=CARTESIAN_POINT('Ctrl Pts',(2.21179541836268,-11.085196814953,107.544320789817));
#47446=CARTESIAN_POINT('Ctrl Pts',(2.20441975696894,-11.,107.490360561254));
#47447=CARTESIAN_POINT('',(2.21863466801864,-9.9,107.59435663812));
#47448=CARTESIAN_POINT('',(2.21863466801864,-11.25,107.59435663812));
#47449=CARTESIAN_POINT('',(2.20441975696895,-9.9,107.490360561254));
#47450=CARTESIAN_POINT('',(2.21863466801864,-9.9,107.59435663812));
#47451=CARTESIAN_POINT('',(2.20441975696895,-10.4,107.490360561254));
#47452=CARTESIAN_POINT('Origin',(2.1284755419274,-9.9,107.508451031791));
#47453=CARTESIAN_POINT('',(2.11375013183874,-9.9,107.598416412742));
#47454=CARTESIAN_POINT('Origin',(3.,-9.9,108.25));
#47455=CARTESIAN_POINT('',(2.03831641583615,-9.9,107.601336231974));
#47456=CARTESIAN_POINT('Origin',(2.03831641583615,-11.25,107.601336231974));
#47457=CARTESIAN_POINT('',(2.11375013183874,-11.,107.598416412742));
#47458=CARTESIAN_POINT('Ctrl Pts',(2.11375013183874,-11.,107.598416412742));
#47459=CARTESIAN_POINT('Ctrl Pts',(2.16817135344136,-11.0851968149524,107.59630992591));
#47460=CARTESIAN_POINT('Ctrl Pts',(2.21863466801864,-11.16,107.59435663812));
#47461=CARTESIAN_POINT('',(2.11375013183874,-10.4,107.598416412742));
#47462=CARTESIAN_POINT('Origin',(2.82287885877973,-11.25,107.245496091928));
#47463=CARTESIAN_POINT('',(2.82287885877973,-11.16,107.245496091928));
#47464=CARTESIAN_POINT('',(2.87883699482611,-11.,107.156693306443));
#47465=CARTESIAN_POINT('Ctrl Pts',(2.82287885877973,-11.16,107.245496091928));
#47466=CARTESIAN_POINT('Ctrl Pts',(2.84980211291508,-11.0851968149532,107.20277022344));
#47467=CARTESIAN_POINT('Ctrl Pts',(2.87883699482611,-11.,107.156693306443));
#47468=CARTESIAN_POINT('',(2.82287885877973,-9.9,107.245496091928));
#47469=CARTESIAN_POINT('',(2.82287885877973,-11.25,107.245496091928));
#47470=CARTESIAN_POINT('',(2.87883699482611,-9.9,107.156693306443));
#47471=CARTESIAN_POINT('',(2.82287885877973,-9.9,107.245496091928));
#47472=CARTESIAN_POINT('',(2.87883699482611,-10.4,107.156693306443));
#47473=CARTESIAN_POINT('Origin',(2.79967157885455,-9.9,107.169160896813));
#47474=CARTESIAN_POINT('',(2.73992306984477,-9.9,107.181187579413));
#47475=CARTESIAN_POINT('Origin',(3.,-9.9,108.25));
#47476=CARTESIAN_POINT('',(2.68026066725228,-9.9,107.134936432712));
#47477=CARTESIAN_POINT('Origin',(2.68026066725228,-11.25,107.134936432712));
#47478=CARTESIAN_POINT('',(2.73992306984477,-11.,107.181187579413));
#47479=CARTESIAN_POINT('Ctrl Pts',(2.73992306984477,-11.,107.181187579413));
#47480=CARTESIAN_POINT('Ctrl Pts',(2.7829661678775,-11.0851968149535,107.214555203831));
#47481=CARTESIAN_POINT('Ctrl Pts',(2.82287885877973,-11.16,107.245496091928));
#47482=CARTESIAN_POINT('',(2.73992306984477,-10.4,107.181187579413));
#47483=CARTESIAN_POINT('Origin',(3.51,-11.25,107.36665408814));
#47484=CARTESIAN_POINT('',(3.51,-11.16,107.36665408814));
#47485=CARTESIAN_POINT('',(3.60994774938095,-11.,107.334596404297));
#47486=CARTESIAN_POINT('Ctrl Pts',(3.51,-11.16,107.36665408814));
#47487=CARTESIAN_POINT('Ctrl Pts',(3.55808806809884,-11.0851968149519,107.351230108178));
#47488=CARTESIAN_POINT('Ctrl Pts',(3.60994774938095,-11.,107.334596404297));
#47489=CARTESIAN_POINT('',(3.51,-9.9,107.36665408814));
#47490=CARTESIAN_POINT('',(3.51,-11.25,107.36665408814));
#47491=CARTESIAN_POINT('',(3.60994774938095,-9.9,107.334596404297));
#47492=CARTESIAN_POINT('',(3.51,-9.9,107.36665408814));
#47493=CARTESIAN_POINT('',(3.60994774938095,-10.4,107.334596404297));
#47494=CARTESIAN_POINT('Origin',(3.5768226993136,-9.9,107.278470678637));
#47495=CARTESIAN_POINT('',(3.48778889390353,-9.9,107.264067956204));
#47496=CARTESIAN_POINT('Origin',(3.,-9.9,108.25));
#47497=CARTESIAN_POINT('',(3.47181450596793,-9.9,107.190287269135));
#47498=CARTESIAN_POINT('Origin',(3.47181450596793,-11.25,107.190287269135));
#47499=CARTESIAN_POINT('',(3.48778889390353,-11.,107.264067956204));
#47500=CARTESIAN_POINT('Ctrl Pts',(3.48778889390353,-11.,107.264067956204));
#47501=CARTESIAN_POINT('Ctrl Pts',(3.49931352442529,-11.0851968149527,107.317296609567));
#47502=CARTESIAN_POINT('Ctrl Pts',(3.51,-11.16,107.36665408814));
#47503=CARTESIAN_POINT('',(3.48778889390353,-10.4,107.264067956204));
#47504=CARTESIAN_POINT('Origin',(3.95848647320163,-11.25,107.901139453808));
#47505=CARTESIAN_POINT('',(3.95848647320163,-11.16,107.901139453808));
#47506=CARTESIAN_POINT('',(4.05565717318629,-11.,107.940827018159));
#47507=CARTESIAN_POINT('Ctrl Pts',(3.95848647320163,-11.16,107.901139453808));
#47508=CARTESIAN_POINT('Ctrl Pts',(4.00523841376049,-11.0851968149523,107.920234414015));
#47509=CARTESIAN_POINT('Ctrl Pts',(4.05565717318629,-11.,107.940827018159));
#47510=CARTESIAN_POINT('',(3.95848647320163,-9.9,107.901139453808));
#47511=CARTESIAN_POINT('',(3.95848647320163,-11.25,107.901139453808));
#47512=CARTESIAN_POINT('',(4.05565717318629,-9.9,107.940827018159));
#47513=CARTESIAN_POINT('',(3.95848647320163,-9.9,107.901139453808));
#47514=CARTESIAN_POINT('',(4.05565717318629,-10.4,107.940827018159));
#47515=CARTESIAN_POINT('Origin',(4.04201475784089,-9.9,107.855430035415));
#47516=CARTESIAN_POINT('',(4.00741287333515,-9.9,107.808276893701));
#47517=CARTESIAN_POINT('Origin',(3.,-9.9,108.25));
#47518=CARTESIAN_POINT('',(4.04260109370703,-9.9,107.741489469725));
#47519=CARTESIAN_POINT('Origin',(4.04260109370703,-11.25,107.741489469725));
#47520=CARTESIAN_POINT('',(4.00741287333515,-11.,107.808276893701));
#47521=CARTESIAN_POINT('Ctrl Pts',(4.00741287333515,-11.,107.808276893701));
#47522=CARTESIAN_POINT('Ctrl Pts',(3.98202653364324,-11.0851968149526,107.85646029753));
#47523=CARTESIAN_POINT('Ctrl Pts',(3.95848647320163,-11.16,107.901139453808));
#47524=CARTESIAN_POINT('',(4.00741287333515,-10.4,107.808276893701));
#47525=CARTESIAN_POINT('Origin',(3.,-10.4,108.25));
#47526=CARTESIAN_POINT('Origin',(3.,-11.,108.25));
#47527=CARTESIAN_POINT('Origin',(3.,-11.,108.25));
#47528=CARTESIAN_POINT('Origin',(3.,-11.,108.25));
#47529=CARTESIAN_POINT('Origin',(3.,-11.,108.25));
#47530=CARTESIAN_POINT('Origin',(3.,-11.,108.25));
#47531=CARTESIAN_POINT('Origin',(3.,-11.,108.25));
#47532=CARTESIAN_POINT('Origin',(3.,-11.,108.25));
#47533=CARTESIAN_POINT('',(1.9,-9.8,108.25));
#47534=CARTESIAN_POINT('',(1.9,-10.4,108.25));
#47535=CARTESIAN_POINT('Origin',(3.,-9.8,108.25));
#47536=CARTESIAN_POINT('Origin',(3.,-11.,108.25));
#47537=CARTESIAN_POINT('Origin',(3.,-11.,108.25));
#47538=CARTESIAN_POINT('Origin',(3.,-11.,108.25));
#47539=CARTESIAN_POINT('Origin',(3.,-11.,108.25));
#47540=CARTESIAN_POINT('Origin',(3.,-11.,108.25));
#47541=CARTESIAN_POINT('Origin',(3.,-11.,108.25));
#47542=CARTESIAN_POINT('Origin',(3.,-11.,108.25));
#47543=CARTESIAN_POINT('Origin',(3.,-11.,108.25));
#47544=CARTESIAN_POINT('Origin',(3.,-11.,108.25));
#47545=CARTESIAN_POINT('Origin',(3.,-11.,108.25));
#47546=CARTESIAN_POINT('Origin',(3.,-11.,108.25));
#47547=CARTESIAN_POINT('Ctrl Pts',(2.85670976047873,-7.7022936971308,108.538667772505));
#47548=CARTESIAN_POINT('Ctrl Pts',(2.80890461182963,-7.70558832612884,108.514938032462));
#47549=CARTESIAN_POINT('Ctrl Pts',(2.72581310601332,-7.71217758412491,108.443301532936));
#47550=CARTESIAN_POINT('Ctrl Pts',(2.64543880465911,-7.72535610011706,108.237507022022));
#47551=CARTESIAN_POINT('Ctrl Pts',(2.75646225010103,-7.74182924510724,107.957765662282));
#47552=CARTESIAN_POINT('Ctrl Pts',(3.11264948697861,-7.76159701909547,107.88639744465));
#47553=CARTESIAN_POINT('Ctrl Pts',(3.36586763099966,-7.78136479308369,108.145991153067));
#47554=CARTESIAN_POINT('Ctrl Pts',(3.2869314131236,-7.80113256707191,108.499845495719));
#47555=CARTESIAN_POINT('Ctrl Pts',(2.9471249283031,-7.82090034106013,108.626779562835));
#47556=CARTESIAN_POINT('Ctrl Pts',(2.65543060635616,-7.84066811504835,108.411277484445));
#47557=CARTESIAN_POINT('Ctrl Pts',(2.67682067977961,-7.86043588903657,108.049245789717));
#47558=CARTESIAN_POINT('Ctrl Pts',(2.99189987276353,-7.88020366302479,107.869629820223));
#47559=CARTESIAN_POINT('Ctrl Pts',(3.31433362603907,-7.89997143701301,108.035664564453));
#47560=CARTESIAN_POINT('Ctrl Pts',(3.35113263206487,-7.91973921100123,108.396465308122));
#47561=CARTESIAN_POINT('Ctrl Pts',(3.06885322266343,-7.93950698498945,108.624172910368));
#47562=CARTESIAN_POINT('Ctrl Pts',(2.72400691454818,-7.95927475897767,108.511865992208));
#47563=CARTESIAN_POINT('Ctrl Pts',(2.62995753252861,-7.9790425329659,108.161599513052));
#47564=CARTESIAN_POINT('Ctrl Pts',(2.87216892550497,-7.99881030695412,107.891663181036));
#47565=CARTESIAN_POINT('Ctrl Pts',(3.23054141520414,-8.01857808094234,107.94735052791));
#47566=CARTESIAN_POINT('Ctrl Pts',(3.37941904127915,-8.03834585493056,108.278057929909));
#47567=CARTESIAN_POINT('Ctrl Pts',(3.18351543540106,-8.05811362891878,108.583268869327));
#47568=CARTESIAN_POINT('Ctrl Pts',(2.82084984167802,-8.07788140290699,108.585635627028));
#47569=CARTESIAN_POINT('Ctrl Pts',(2.62097947544604,-8.09764917689522,108.283007517633));
#47570=CARTESIAN_POINT('Ctrl Pts',(2.7655281947484,-8.11741695088344,107.950385203063));
#47571=CARTESIAN_POINT('Ctrl Pts',(3.12314338152363,-8.13718472487166,107.890025332106));
#47572=CARTESIAN_POINT('Ctrl Pts',(3.36885715962375,-8.15695249885988,108.156777417877));
#47573=CARTESIAN_POINT('Ctrl Pts',(3.27938738699594,-8.1767202728481,108.508241634873));
#47574=CARTESIAN_POINT('Ctrl Pts',(2.93603598591862,-8.19648804683633,108.625039543106));
#47575=CARTESIAN_POINT('Ctrl Pts',(2.65080921325911,-8.21625582082455,108.401035917761));
#47576=CARTESIAN_POINT('Ctrl Pts',(2.68289499558652,-8.23602359481276,108.039784705191));
#47577=CARTESIAN_POINT('Ctrl Pts',(3.00313671720263,-8.25579136880099,107.869557869052));
#47578=CARTESIAN_POINT('Ctrl Pts',(3.32052807796508,-8.2755591427892,108.045041942749));
#47579=CARTESIAN_POINT('Ctrl Pts',(3.34665292419479,-8.29532691677743,108.406773097638));
#47580=CARTESIAN_POINT('Ctrl Pts',(3.05777139212753,-8.31509469076565,108.626043242523));
#47581=CARTESIAN_POINT('Ctrl Pts',(2.71639251838735,-8.33486246475387,108.503599783851));
#47582=CARTESIAN_POINT('Ctrl Pts',(2.63273010801875,-8.35463023874209,108.150708104863));
#47583=CARTESIAN_POINT('Ctrl Pts',(2.88280888503356,-8.37439801273031,107.888043791918));
#47584=CARTESIAN_POINT('Ctrl Pts',(3.23938019713941,-8.39416578671853,107.954292077865));
#47585=CARTESIAN_POINT('Ctrl Pts',(3.37842474494008,-8.41393356070675,108.289252597531));
#47586=CARTESIAN_POINT('Ctrl Pts',(3.17359159824674,-8.43370133469497,108.588543957285));
#47587=CARTESIAN_POINT('Ctrl Pts',(2.81101433099364,-8.45346910868319,108.580197624016));
#47588=CARTESIAN_POINT('Ctrl Pts',(2.62016990367575,-8.47323688267142,108.271797979773));
#47589=CARTESIAN_POINT('Ctrl Pts',(2.77448022527394,-8.49300465665964,107.943590331087));
#47590=CARTESIAN_POINT('Ctrl Pts',(3.1337222307341,-8.51277243064786,107.893819681898));
#47591=CARTESIAN_POINT('Ctrl Pts',(3.37144973952803,-8.53254020463607,108.167713032621));
#47592=CARTESIAN_POINT('Ctrl Pts',(3.27163779891431,-8.5523079786243,108.51638123094));
#47593=CARTESIAN_POINT('Ctrl Pts',(2.92498634456088,-8.57207575261252,108.622986602298));
#47594=CARTESIAN_POINT('Ctrl Pts',(2.6465004191082,-8.59184352660074,108.390655964343));
#47595=CARTESIAN_POINT('Ctrl Pts',(2.68924248550083,-8.61161130058896,108.030510088664));
#47596=CARTESIAN_POINT('Ctrl Pts',(3.01437247462189,-8.63137907457718,107.869816510131));
#47597=CARTESIAN_POINT('Ctrl Pts',(3.32644207722428,-8.6511468485654,108.05459881215));
#47598=CARTESIAN_POINT('Ctrl Pts',(3.34187106527198,-8.67091462255362,108.41694378912));
#47599=CARTESIAN_POINT('Ctrl Pts',(3.04663898976117,-8.69068239654184,108.627585564647));
#47600=CARTESIAN_POINT('Ctrl Pts',(2.70902567864924,-8.71045017053006,108.495112215751));
#47601=CARTESIAN_POINT('Ctrl Pts',(2.63582313908689,-8.73021794451829,108.139903369846));
#47602=CARTESIAN_POINT('Ctrl Pts',(2.89355112400359,-8.7499857185065,107.884740242026));
#47603=CARTESIAN_POINT('Ctrl Pts',(3.2480100826438,-8.76975349249473,107.961491676198));
#47604=CARTESIAN_POINT('Ctrl Pts',(3.37710022867022,-8.78952126648294,108.300413009558));
#47605=CARTESIAN_POINT('Ctrl Pts',(3.16351627908797,-8.80928904047117,108.593523624325));
#47606=CARTESIAN_POINT('Ctrl Pts',(2.80134373476698,-8.82905681445938,108.574471481458));
#47607=CARTESIAN_POINT('Ctrl Pts',(2.6196917811276,-8.84882458844761,108.260569420702));
#47608=CARTESIAN_POINT('Ctrl Pts',(2.78362905031687,-8.86859236243583,107.937062839968));
#47609=CARTESIAN_POINT('Ctrl Pts',(3.14418439041029,-8.88836013642405,107.897924843879));
#47610=CARTESIAN_POINT('Ctrl Pts',(3.37371818283995,-8.90812791041227,108.178720453069));
#47611=CARTESIAN_POINT('Ctrl Pts',(3.26365117266921,-8.9278956844005,108.524288375886));
#47612=CARTESIAN_POINT('Ctrl Pts',(2.91400216206011,-8.94766345838871,108.620608183754));
#47613=CARTESIAN_POINT('Ctrl Pts',(2.64250009780596,-8.96743123237694,108.380153270904));
#47614=CARTESIAN_POINT('Ctrl Pts',(2.69586115043873,-8.98719900636515,108.021427004694));
#47615=CARTESIAN_POINT('Ctrl Pts',(3.02559569024832,-9.00696678035338,107.87040690913));
#47616=CARTESIAN_POINT('Ctrl Pts',(3.332071214708,-9.02673455434159,108.064326193666));
#47617=CARTESIAN_POINT('Ctrl Pts',(3.33679088083925,-9.04650232832982,108.426968801146));
#47618=CARTESIAN_POINT('Ctrl Pts',(3.03546588901117,-9.06627010231804,108.628798395868));
#47619=CARTESIAN_POINT('Ctrl Pts',(2.70191275060503,-9.08603787630626,108.486410756411));
#47620=CARTESIAN_POINT('Ctrl Pts',(2.63923396028456,-9.10580565029448,108.129194707984));
#47621=CARTESIAN_POINT('Ctrl Pts',(2.90438625299112,-9.1255734242827,107.881755427227));
#47622=CARTESIAN_POINT('Ctrl Pts',(3.2564235481909,-9.14534119827092,107.968943034321));
#47623=CARTESIAN_POINT('Ctrl Pts',(3.37544664493324,-9.16510897225914,108.311529429926));
#47624=CARTESIAN_POINT('Ctrl Pts',(3.15329827158403,-9.18487674624737,108.59820352372));
#47625=CARTESIAN_POINT('Ctrl Pts',(2.79184649073512,-9.20464452023558,108.568462196868));
#47626=CARTESIAN_POINT('Ctrl Pts',(2.61954552618002,-9.22441229422381,108.249331638151));
#47627=CARTESIAN_POINT('Ctrl Pts',(2.7929666844032,-9.24418006821203,107.930808426606));
#47628=CARTESIAN_POINT('Ctrl Pts',(3.15452073504689,-9.26394784220025,107.902337234153));
#47629=CARTESIAN_POINT('Ctrl Pts',(3.37566050136972,-9.28371561618847,108.1897900773));
#47630=CARTESIAN_POINT('Ctrl Pts',(3.25543449645413,-9.30348339017669,108.531956162289));
#47631=CARTESIAN_POINT('Ctrl Pts',(2.90309298249399,-9.32325116416491,108.617906379101));
#47632=CARTESIAN_POINT('Ctrl Pts',(2.63881182940184,-9.34301893815313,108.369536967137));
#47633=CARTESIAN_POINT('Ctrl Pts',(2.70274502066785,-9.36278671214135,108.012543455793));
#47634=CARTESIAN_POINT('Ctrl Pts',(3.03679699339086,-9.38255448612957,107.871328383607));
#47635=CARTESIAN_POINT('Ctrl Pts',(3.3374096596431,-9.40232226011779,108.074215959287));
#47636=CARTESIAN_POINT('Ctrl Pts',(3.33141880989063,-9.42209003410602,108.436838588562));
#47637=CARTESIAN_POINT('Ctrl Pts',(3.0242574980433,-9.44185780809423,108.629682366924));
#47638=CARTESIAN_POINT('Ctrl Pts',(2.69506947405166,-9.46162558208246,108.477499161251));
#47639=CARTESIAN_POINT('Ctrl Pts',(2.64293914677449,-9.48139335607067,108.11859924174));
#47640=CARTESIAN_POINT('Ctrl Pts',(2.91535037624978,-9.50116113005889,107.879072987278));
#47641=CARTESIAN_POINT('Ctrl Pts',(3.26451785003709,-9.52092890404712,107.976673691963));
#47642=CARTESIAN_POINT('Ctrl Pts',(3.37368648223413,-9.54069667803533,108.322492331795));
#47643=CARTESIAN_POINT('Ctrl Pts',(3.1425103302508,-9.56046445202356,108.602707172509));
#47644=CARTESIAN_POINT('Ctrl Pts',(2.84350450152926,-9.57693759701374,108.568400494187));
#47645=CARTESIAN_POINT('Ctrl Pts',(2.70009555898594,-9.59011611300589,108.400337160175));
#47646=CARTESIAN_POINT('Ctrl Pts',(2.67621270542783,-9.59670537100196,108.293259638215));
#47647=CARTESIAN_POINT('Ctrl Pts',(2.67788283232033,-9.6,108.239915065145));
#47648=CARTESIAN_POINT('Ctrl Pts',(2.84618335780813,-7.71596246475387,108.559873914818));
#47649=CARTESIAN_POINT('Ctrl Pts',(2.79486634229295,-7.71925709375191,108.534400938113));
#47650=CARTESIAN_POINT('Ctrl Pts',(2.7056707595231,-7.72584635174798,108.457501870512));
#47651=CARTESIAN_POINT('Ctrl Pts',(2.61939199277579,-7.73902486774013,108.236589261557));
#47652=CARTESIAN_POINT('Ctrl Pts',(2.73857145426251,-7.75549801273031,107.936297512579));
#47653=CARTESIAN_POINT('Ctrl Pts',(3.12092495545807,-7.77526578671853,107.859686435425));
#47654=CARTESIAN_POINT('Ctrl Pts',(3.39274503745041,-7.79503356070675,108.138350444197));
#47655=CARTESIAN_POINT('Ctrl Pts',(3.30800999882123,-7.81480133469497,108.518199671845));
#47656=CARTESIAN_POINT('Ctrl Pts',(2.94324061421599,-7.8345691086832,108.654458582772));
#47657=CARTESIAN_POINT('Ctrl Pts',(2.6301178132617,-7.85433688267141,108.423125267997));
#47658=CARTESIAN_POINT('Ctrl Pts',(2.65307924651231,-7.87410465665964,108.034497962773));
#47659=CARTESIAN_POINT('Ctrl Pts',(2.99130482036317,-7.89387243064785,107.841687026006));
#47660=CARTESIAN_POINT('Ctrl Pts',(3.33742523598857,-7.91364020463608,108.019919032108));
#47661=CARTESIAN_POINT('Ctrl Pts',(3.37692757447162,-7.9334079786243,108.407224958017));
#47662=CARTESIAN_POINT('Ctrl Pts',(3.07391132536006,-7.95317575261252,108.651660440127));
#47663=CARTESIAN_POINT('Ctrl Pts',(2.70373188143028,-7.97294352660074,108.531103219314));
#47664=CARTESIAN_POINT('Ctrl Pts',(2.60277343380117,-7.99271130058896,108.155105427167));
#47665=CARTESIAN_POINT('Ctrl Pts',(2.86277818564407,-8.01247907457718,107.865339003892));
#47666=CARTESIAN_POINT('Ctrl Pts',(3.2474774729342,-8.0322468485654,107.925117260508));
#47667=CARTESIAN_POINT('Ctrl Pts',(3.40729196285943,-8.05201462255362,108.280119124511));
#47668=CARTESIAN_POINT('Ctrl Pts',(3.1969968656489,-8.07178239654184,108.607751502113));
#47669=CARTESIAN_POINT('Ctrl Pts',(2.80768909387483,-8.09155017053006,108.610292126818));
#47670=CARTESIAN_POINT('Ctrl Pts',(2.59313582974341,-8.11131794451828,108.28543231937));
#47671=CARTESIAN_POINT('Ctrl Pts',(2.74830340229062,-8.13108571850651,107.928374869287));
#47672=CARTESIAN_POINT('Ctrl Pts',(3.13218975358964,-8.15085349249472,107.863580835131));
#47673=CARTESIAN_POINT('Ctrl Pts',(3.39595418314122,-8.17062126648295,108.149929090729));
#47674=CARTESIAN_POINT('Ctrl Pts',(3.29991177265145,-8.19038904047117,108.527212609058));
#47675=CARTESIAN_POINT('Ctrl Pts',(2.9313370547779,-8.21015681445939,108.652590737531));
#47676=CARTESIAN_POINT('Ctrl Pts',(2.62515692289811,-8.22992458844761,108.412131334263));
#47677=CARTESIAN_POINT('Ctrl Pts',(2.65959979434693,-8.24969236243583,108.024341847059));
#47678=CARTESIAN_POINT('Ctrl Pts',(3.0033671470522,-8.26946013642405,107.84160978915));
#47679=CARTESIAN_POINT('Ctrl Pts',(3.34407474539452,-8.28922791041227,108.029985292356));
#47680=CARTESIAN_POINT('Ctrl Pts',(3.37211877783007,-8.30899568440049,108.418289979452));
#47681=CARTESIAN_POINT('Ctrl Pts',(3.06201540022193,-8.32876345838871,108.65366817082));
#47682=CARTESIAN_POINT('Ctrl Pts',(2.69555811569654,-8.34853123237693,108.522229757888));
#47683=CARTESIAN_POINT('Ctrl Pts',(2.60574968852405,-8.36829900636515,108.143413913202));
#47684=CARTESIAN_POINT('Ctrl Pts',(2.87419977900041,-8.38806678035338,107.86145372683));
#47685=CARTESIAN_POINT('Ctrl Pts',(3.25696557039913,-8.4078345543416,107.932568751338));
#47686=CARTESIAN_POINT('Ctrl Pts',(3.40622462341796,-8.42760232832982,108.292136175986));
#47687=CARTESIAN_POINT('Ctrl Pts',(3.18634400252412,-8.44737010231804,108.613414109139));
#47688=CARTESIAN_POINT('Ctrl Pts',(2.79713104586844,-8.46713787630626,108.604454636657));
#47689=CARTESIAN_POINT('Ctrl Pts',(2.59226678512645,-8.48690565029448,108.273399305259));
#47690=CARTESIAN_POINT('Ctrl Pts',(2.75791306782568,-8.5066734242827,107.921080831711));
#47691=CARTESIAN_POINT('Ctrl Pts',(3.14354574733523,-8.52644119827092,107.867653925848));
#47692=CARTESIAN_POINT('Ctrl Pts',(3.39873721942354,-8.54620897225914,108.161668058755));
#47693=CARTESIAN_POINT('Ctrl Pts',(3.29159288351379,-8.56597674624736,108.535950156989));
#47694=CARTESIAN_POINT('Ctrl Pts',(2.91947568350271,-8.58574452023558,108.650386983368));
#47695=CARTESIAN_POINT('Ctrl Pts',(2.62053159565738,-8.6055122942238,108.400988847613));
#47696=CARTESIAN_POINT('Ctrl Pts',(2.666413584234,-8.62528006821202,108.014385897676));
#47697=CARTESIAN_POINT('Ctrl Pts',(3.01542830686663,-8.64504784220025,107.841887430548));
#47698=CARTESIAN_POINT('Ctrl Pts',(3.35042319949031,-8.66481561618847,108.040244229503));
#47699=CARTESIAN_POINT('Ctrl Pts',(3.36698563348334,-8.68458339017668,108.429207831343));
#47700=CARTESIAN_POINT('Ctrl Pts',(3.05006518814019,-8.70435116416491,108.655323795174));
#47701=CARTESIAN_POINT('Ctrl Pts',(2.68765009240153,-8.72411893815312,108.513118675166));
#47702=CARTESIAN_POINT('Ctrl Pts',(2.60906994016635,-8.74388671214136,108.131815439603));
#47703=CARTESIAN_POINT('Ctrl Pts',(2.8857311654613,-8.76365448612956,107.857907491208));
#47704=CARTESIAN_POINT('Ctrl Pts',(3.26622942546156,-8.78342226011779,107.940297247322));
#47705=CARTESIAN_POINT('Ctrl Pts',(3.40480280539435,-8.80319003410601,108.304116455377));
#47706=CARTESIAN_POINT('Ctrl Pts',(3.17552852920793,-8.82295780809423,108.618759593003));
#47707=CARTESIAN_POINT('Ctrl Pts',(2.78675002728303,-8.84272558208245,108.59830783961));
#47708=CARTESIAN_POINT('Ctrl Pts',(2.5917535386893,-8.86249335607067,108.261345872599));
#47709=CARTESIAN_POINT('Ctrl Pts',(2.76773398481769,-8.8822611300589,107.914073817351));
#47710=CARTESIAN_POINT('Ctrl Pts',(3.15477647928768,-8.90202890404711,107.87206066167));
#47711=CARTESIAN_POINT('Ctrl Pts',(3.40117230735701,-8.92179667803534,108.173484107483));
#47712=CARTESIAN_POINT('Ctrl Pts',(3.28301954289012,-8.94156445202356,108.54443817745));
#47713=CARTESIAN_POINT('Ctrl Pts',(2.90768457982995,-8.96133222601178,108.647833841191));
#47714=CARTESIAN_POINT('Ctrl Pts',(2.61623740233022,-8.98109999999999,108.389714604203));
#47715=CARTESIAN_POINT('Ctrl Pts',(2.67351847023281,-9.00086777398822,108.004635551233));
#47716=CARTESIAN_POINT('Ctrl Pts',(3.02747600354171,-9.02063554797644,107.8425212015));
#47717=CARTESIAN_POINT('Ctrl Pts',(3.35646586526486,-9.04040332196466,108.050686204945));
#47718=CARTESIAN_POINT('Ctrl Pts',(3.36153224800663,-9.06017109595288,108.439969301858));
#47719=CARTESIAN_POINT('Ctrl Pts',(3.03807128788586,-9.0799388699411,108.65662572353));
#47720=CARTESIAN_POINT('Ctrl Pts',(2.68001463368803,-9.09970664392932,108.503777988303));
#47721=CARTESIAN_POINT('Ctrl Pts',(2.61273132747015,-9.11947441791754,108.120320096896));
#47722=CARTESIAN_POINT('Ctrl Pts',(2.89736226583594,-9.13924219190577,107.854703405629));
#47723=CARTESIAN_POINT('Ctrl Pts',(3.27526096190099,-9.15900996589399,107.948295997901));
#47724=CARTESIAN_POINT('Ctrl Pts',(3.40302774591469,-9.17877773988221,108.316049511389));
#47725=CARTESIAN_POINT('Ctrl Pts',(3.16455988536032,-9.19854551387043,108.623783287661));
#47726=CARTESIAN_POINT('Ctrl Pts',(2.77655509570962,-9.21831328785865,108.591857100323));
#47727=CARTESIAN_POINT('Ctrl Pts',(2.59159653954535,-9.23808106184686,108.249282538883));
#47728=CARTESIAN_POINT('Ctrl Pts',(2.77775758116294,-9.25784883583509,107.907359941616));
#47729=CARTESIAN_POINT('Ctrl Pts',(3.16587215356286,-9.27761660982331,107.876797195424));
#47730=CARTESIAN_POINT('Ctrl Pts',(3.40325731269523,-9.29738438381153,108.185366929616));
#47731=CARTESIAN_POINT('Ctrl Pts',(3.27419925234135,-9.31715215779975,108.552669255586));
#47732=CARTESIAN_POINT('Ctrl Pts',(2.89597398896532,-9.33691993178797,108.644933556279));
#47733=CARTESIAN_POINT('Ctrl Pts',(2.61227818596405,-9.3566877057762,108.37831840441));
#47734=CARTESIAN_POINT('Ctrl Pts',(2.68090804406188,-9.37645547976442,107.995099398128));
#47735=CARTESIAN_POINT('Ctrl Pts',(3.03950017799571,-9.39622325375263,107.843510369433));
#47736=CARTESIAN_POINT('Ctrl Pts',(3.36219648360416,-9.41599102774086,108.06130249357));
#47737=CARTESIAN_POINT('Ctrl Pts',(3.35576553341607,-9.43575880172908,108.450564144638));
#47738=CARTESIAN_POINT('Ctrl Pts',(3.02603950491996,-9.4555265757173,108.657574632961));
#47739=CARTESIAN_POINT('Ctrl Pts',(2.67266863563159,-9.47529434970552,108.4942117286));
#47740=CARTESIAN_POINT('Ctrl Pts',(2.61670870476033,-9.49506212369374,108.108946265394));
#47741=CARTESIAN_POINT('Ctrl Pts',(2.90913183667244,-9.51482989768196,107.851823907994));
#47742=CARTESIAN_POINT('Ctrl Pts',(3.28394988820209,-9.53459767167018,107.956594565928));
#47743=CARTESIAN_POINT('Ctrl Pts',(3.40113827795794,-9.5543654456584,108.32781777111));
#47744=CARTESIAN_POINT('Ctrl Pts',(3.15297943914441,-9.57413321964662,108.628617783972));
#47745=CARTESIAN_POINT('Ctrl Pts',(2.83200801273462,-9.59060636463681,108.591790864833));
#47746=CARTESIAN_POINT('Ctrl Pts',(2.67806394734679,-9.60378488062895,108.411381244473));
#47747=CARTESIAN_POINT('Ctrl Pts',(2.65242660908466,-9.61037413862503,108.296437582315));
#47748=CARTESIAN_POINT('Ctrl Pts',(2.65421942701488,-9.61366876762306,108.239174204598));
#47749=CARTESIAN_POINT('Ctrl Pts',(2.83565695513754,-7.72963123237693,108.581080057132));
#47750=CARTESIAN_POINT('Ctrl Pts',(2.78082807275627,-7.73292586137497,108.553863843763));
#47751=CARTESIAN_POINT('Ctrl Pts',(2.68552841303288,-7.73951511937104,108.471702208088));
#47752=CARTESIAN_POINT('Ctrl Pts',(2.59334518089247,-7.75269363536319,108.235671501093));
#47753=CARTESIAN_POINT('Ctrl Pts',(2.72068065842399,-7.76916678035337,107.914829362876));
#47754=CARTESIAN_POINT('Ctrl Pts',(3.12920042393753,-7.78893455434159,107.832975426201));
#47755=CARTESIAN_POINT('Ctrl Pts',(3.41962244390117,-7.80870232832982,108.130709735327));
#47756=CARTESIAN_POINT('Ctrl Pts',(3.32908858451885,-7.82847010231803,108.536553847972));
#47757=CARTESIAN_POINT('Ctrl Pts',(2.93935630012888,-7.84823787630626,108.682137602709));
#47758=CARTESIAN_POINT('Ctrl Pts',(2.60480502016724,-7.86800565029448,108.434973051549));
#47759=CARTESIAN_POINT('Ctrl Pts',(2.62933781324501,-7.8877734242827,108.019750135828));
#47760=CARTESIAN_POINT('Ctrl Pts',(2.99070976796282,-7.90754119827092,107.813744231789));
#47761=CARTESIAN_POINT('Ctrl Pts',(3.36051684593806,-7.92730897225914,108.004173499763));
#47762=CARTESIAN_POINT('Ctrl Pts',(3.40272251687838,-7.94707674624736,108.417984607911));
#47763=CARTESIAN_POINT('Ctrl Pts',(3.07896942805669,-7.96684452023559,108.679147969885));
#47764=CARTESIAN_POINT('Ctrl Pts',(2.68345684831238,-7.9866122942238,108.55034044642));
#47765=CARTESIAN_POINT('Ctrl Pts',(2.57558933507373,-8.00638006821202,108.148611341282));
#47766=CARTESIAN_POINT('Ctrl Pts',(2.85338744578317,-8.02614784220024,107.839014826749));
#47767=CARTESIAN_POINT('Ctrl Pts',(3.26441353066427,-8.04591561618847,107.902883993107));
#47768=CARTESIAN_POINT('Ctrl Pts',(3.43516488443971,-8.06568339017668,108.282180319114));
#47769=CARTESIAN_POINT('Ctrl Pts',(3.21047829589673,-8.08545116416491,108.6322341349));
#47770=CARTESIAN_POINT('Ctrl Pts',(2.79452834607165,-8.10521893815313,108.634948626608));
#47771=CARTESIAN_POINT('Ctrl Pts',(2.56529218404078,-8.12498671214135,108.287857121108));
#47772=CARTESIAN_POINT('Ctrl Pts',(2.73107860983284,-8.14475448612956,107.906364535512));
#47773=CARTESIAN_POINT('Ctrl Pts',(3.14123612565564,-8.16452226011779,107.837136338157));
#47774=CARTESIAN_POINT('Ctrl Pts',(3.42305120665869,-8.18429003410601,108.14308076358));
#47775=CARTESIAN_POINT('Ctrl Pts',(3.32043615830696,-8.20405780809423,108.546183583244));
#47776=CARTESIAN_POINT('Ctrl Pts',(2.92663812363718,-8.22382558208245,108.680141931955));
#47777=CARTESIAN_POINT('Ctrl Pts',(2.59950463253712,-8.24359335607067,108.423226750764));
#47778=CARTESIAN_POINT('Ctrl Pts',(2.63630459310734,-8.26336113005889,108.008898988927));
#47779=CARTESIAN_POINT('Ctrl Pts',(3.00359757690178,-8.28312890404712,107.813661709249));
#47780=CARTESIAN_POINT('Ctrl Pts',(3.36762141282396,-8.30289667803533,108.014928641963));
#47781=CARTESIAN_POINT('Ctrl Pts',(3.39758463146536,-8.32266445202356,108.429806861266));
#47782=CARTESIAN_POINT('Ctrl Pts',(3.06625940831632,-8.34243222601178,108.681293099116));
#47783=CARTESIAN_POINT('Ctrl Pts',(2.67472371300574,-8.3622,108.540859731924));
#47784=CARTESIAN_POINT('Ctrl Pts',(2.57876926902934,-8.38196777398822,108.136119721542));
#47785=CARTESIAN_POINT('Ctrl Pts',(2.86559067296727,-8.40173554797644,107.834863661742));
#47786=CARTESIAN_POINT('Ctrl Pts',(3.27455094365884,-8.42150332196466,107.910845424811));
#47787=CARTESIAN_POINT('Ctrl Pts',(3.43402450189583,-8.44127109595287,108.29501975444));
#47788=CARTESIAN_POINT('Ctrl Pts',(3.1990964068015,-8.4610388699411,108.638284260993));
#47789=CARTESIAN_POINT('Ctrl Pts',(2.78324776074323,-8.48080664392932,108.628711649297));
#47790=CARTESIAN_POINT('Ctrl Pts',(2.56436366657715,-8.50057441791754,108.275000630746));
#47791=CARTESIAN_POINT('Ctrl Pts',(2.74134591037741,-8.52034219190576,107.898571332334));
#47792=CARTESIAN_POINT('Ctrl Pts',(3.15336926393636,-8.54010996589398,107.841488169797));
#47793=CARTESIAN_POINT('Ctrl Pts',(3.42602469931906,-8.55987773988221,108.155623084889));
#47794=CARTESIAN_POINT('Ctrl Pts',(3.31154796811327,-8.57964551387043,108.555519083038));
#47795=CARTESIAN_POINT('Ctrl Pts',(2.91396502244455,-8.59941328785865,108.677787364438));
#47796=CARTESIAN_POINT('Ctrl Pts',(2.59456277220656,-8.61918106184687,108.411321730883));
#47797=CARTESIAN_POINT('Ctrl Pts',(2.64358468296716,-8.63894883583509,107.998261706687));
#47798=CARTESIAN_POINT('Ctrl Pts',(3.01648413911137,-8.65871660982331,107.813958350965));
#47799=CARTESIAN_POINT('Ctrl Pts',(3.37440432175633,-8.67848438381153,108.025889646857));
#47800=CARTESIAN_POINT('Ctrl Pts',(3.39210020169469,-8.69825215779975,108.441471873566));
#47801=CARTESIAN_POINT('Ctrl Pts',(3.0534913865192,-8.71801993178797,108.683062025701));
#47802=CARTESIAN_POINT('Ctrl Pts',(2.66627450615383,-8.73778770577619,108.531125134581));
#47803=CARTESIAN_POINT('Ctrl Pts',(2.5823167412458,-8.75755547976442,108.123727509361));
#47804=CARTESIAN_POINT('Ctrl Pts',(2.87791120691902,-8.77732325375263,107.831074740389));
#47805=CARTESIAN_POINT('Ctrl Pts',(3.28444876827931,-8.79709102774086,107.919102818446));
#47806=CARTESIAN_POINT('Ctrl Pts',(3.43250538211848,-8.81685880172908,108.307819901196));
#47807=CARTESIAN_POINT('Ctrl Pts',(3.18754077932788,-8.8366265757173,108.643995561682));
#47808=CARTESIAN_POINT('Ctrl Pts',(2.77215631979907,-8.85639434970551,108.622144197762));
#47809=CARTESIAN_POINT('Ctrl Pts',(2.563815296251,-8.87616212369374,108.262122324496));
#47810=CARTESIAN_POINT('Ctrl Pts',(2.7518389193185,-8.89592989768196,107.891084794735));
#47811=CARTESIAN_POINT('Ctrl Pts',(3.16536856816508,-8.91569767167018,107.846196479462));
#47812=CARTESIAN_POINT('Ctrl Pts',(3.42862643187407,-8.9354654456584,108.168247761898));
#47813=CARTESIAN_POINT('Ctrl Pts',(3.30238791311104,-8.95523321964662,108.564587979014));
#47814=CARTESIAN_POINT('Ctrl Pts',(2.90136699759978,-8.97500099363484,108.675059498627));
#47815=CARTESIAN_POINT('Ctrl Pts',(2.58997470685448,-8.99476876762306,108.399275937501));
#47816=CARTESIAN_POINT('Ctrl Pts',(2.65117579002688,-9.01453654161128,107.987844097773));
#47817=CARTESIAN_POINT('Ctrl Pts',(3.02935631683511,-9.0343043155995,107.81463549387));
#47818=CARTESIAN_POINT('Ctrl Pts',(3.38086051582172,-9.05407208958773,108.037046216225));
#47819=CARTESIAN_POINT('Ctrl Pts',(3.38627361517402,-9.07383986357594,108.452969802571));
#47820=CARTESIAN_POINT('Ctrl Pts',(3.04067668676055,-9.09360763756417,108.684453051191));
#47821=CARTESIAN_POINT('Ctrl Pts',(2.65811651677103,-9.11337541155238,108.521145220195));
#47822=CARTESIAN_POINT('Ctrl Pts',(2.58622869465574,-9.13314318554061,108.111445485808));
#47823=CARTESIAN_POINT('Ctrl Pts',(2.89033827868075,-9.15291095952883,107.827651384031));
#47824=CARTESIAN_POINT('Ctrl Pts',(3.29409837561108,-9.17267873351704,107.92764896148));
#47825=CARTESIAN_POINT('Ctrl Pts',(3.43060884689613,-9.19244650750527,108.320569592852));
#47826=CARTESIAN_POINT('Ctrl Pts',(3.17582149913661,-9.21221428149349,108.649363051602));
#47827=CARTESIAN_POINT('Ctrl Pts',(2.76126370068411,-9.23198205548171,108.615252003778));
#47828=CARTESIAN_POINT('Ctrl Pts',(2.56364755291068,-9.25174982946993,108.249233439614));
#47829=CARTESIAN_POINT('Ctrl Pts',(2.76254847792268,-9.27151760345816,107.883911456626));
#47830=CARTESIAN_POINT('Ctrl Pts',(3.17722357207883,-9.29128537744637,107.851257156695));
#47831=CARTESIAN_POINT('Ctrl Pts',(3.43085412402073,-9.3110531514346,108.180943781931));
#47832=CARTESIAN_POINT('Ctrl Pts',(3.29296400822856,-9.33082092542282,108.573382348883));
#47833=CARTESIAN_POINT('Ctrl Pts',(2.88885499543664,-9.35058869941104,108.671960733458));
#47834=CARTESIAN_POINT('Ctrl Pts',(2.58574454252627,-9.37035647339926,108.387099841682));
#47835=CARTESIAN_POINT('Ctrl Pts',(2.65907106745591,-9.39012424738748,107.977655340462));
#47836=CARTESIAN_POINT('Ctrl Pts',(3.04220336260056,-9.4098920213757,107.815692355258));
#47837=CARTESIAN_POINT('Ctrl Pts',(3.38698330756522,-9.42965979536392,108.048389027853));
#47838=CARTESIAN_POINT('Ctrl Pts',(3.38011225694151,-9.44942756935214,108.464289700713));
#47839=CARTESIAN_POINT('Ctrl Pts',(3.02782151179663,-9.46919534334036,108.685466898997));
#47840=CARTESIAN_POINT('Ctrl Pts',(2.65026779721153,-9.48896311732858,108.51092429595));
#47841=CARTESIAN_POINT('Ctrl Pts',(2.59047826274616,-9.5087308913168,108.099293289049));
#47842=CARTESIAN_POINT('Ctrl Pts',(2.9029132970951,-9.52849866530502,107.82457482871));
#47843=CARTESIAN_POINT('Ctrl Pts',(3.3033819263671,-9.54826643929324,107.936515439893));
#47844=CARTESIAN_POINT('Ctrl Pts',(3.42859007368176,-9.56803421328147,108.333143210425));
#47845=CARTESIAN_POINT('Ctrl Pts',(3.16344854803802,-9.58780198726968,108.654528395435));
#47846=CARTESIAN_POINT('Ctrl Pts',(2.82051152393997,-9.60427513225987,108.615181235479));
#47847=CARTESIAN_POINT('Ctrl Pts',(2.65603233570764,-9.61745364825201,108.422425328771));
#47848=CARTESIAN_POINT('Ctrl Pts',(2.62864051274149,-9.62404290624809,108.299615526415));
#47849=CARTESIAN_POINT('Ctrl Pts',(2.63055602170942,-9.62733753524613,108.238433344052));
#47850=CARTESIAN_POINT('Ctrl Pts',(2.82513055246694,-7.7433,108.602286199445));
#47851=CARTESIAN_POINT('Ctrl Pts',(2.7667898032196,-7.74659462899803,108.573326749414));
#47852=CARTESIAN_POINT('Ctrl Pts',(2.66538606654267,-7.75318388699411,108.485902545664));
#47853=CARTESIAN_POINT('Ctrl Pts',(2.56729836900916,-7.76636240298626,108.234753740629));
#47854=CARTESIAN_POINT('Ctrl Pts',(2.70278986258547,-7.78283554797643,107.893361213173));
#47855=CARTESIAN_POINT('Ctrl Pts',(3.13747589241699,-7.80260332196466,107.806264416976));
#47856=CARTESIAN_POINT('Ctrl Pts',(3.44649985035192,-7.82237109595288,108.123069026457));
#47857=CARTESIAN_POINT('Ctrl Pts',(3.35016717021648,-7.8421388699411,108.554908024098));
#47858=CARTESIAN_POINT('Ctrl Pts',(2.93547198604177,-7.86190664392932,108.709816622646));
#47859=CARTESIAN_POINT('Ctrl Pts',(2.57949222707278,-7.88167441791754,108.446820835101));
#47860=CARTESIAN_POINT('Ctrl Pts',(2.60559637997771,-7.90144219190577,108.005002308884));
#47861=CARTESIAN_POINT('Ctrl Pts',(2.99011471556246,-7.92120996589398,107.785801437572));
#47862=CARTESIAN_POINT('Ctrl Pts',(3.38360845588756,-7.94097773988221,107.988427967418));
#47863=CARTESIAN_POINT('Ctrl Pts',(3.42851745928513,-7.96074551387042,108.428744257806));
#47864=CARTESIAN_POINT('Ctrl Pts',(3.08402753075333,-7.98051328785865,108.706635499644));
#47865=CARTESIAN_POINT('Ctrl Pts',(2.66318181519447,-8.00028106184687,108.569577673526));
#47866=CARTESIAN_POINT('Ctrl Pts',(2.54840523634629,-8.02004883583509,108.142117255398));
#47867=CARTESIAN_POINT('Ctrl Pts',(2.84399670592228,-8.03981660982331,107.812690649605));
#47868=CARTESIAN_POINT('Ctrl Pts',(3.28134958839434,-8.05958438381153,107.880650725706));
#47869=CARTESIAN_POINT('Ctrl Pts',(3.46303780601998,-8.07935215779975,108.284241513717));
#47870=CARTESIAN_POINT('Ctrl Pts',(3.22395972614457,-8.09911993178797,108.656716767687));
#47871=CARTESIAN_POINT('Ctrl Pts',(2.78136759826846,-8.11888770577619,108.659605126398));
#47872=CARTESIAN_POINT('Ctrl Pts',(2.53744853833815,-8.13865547976441,108.290281922845));
#47873=CARTESIAN_POINT('Ctrl Pts',(2.71385381737505,-8.15842325375263,107.884354201737));
#47874=CARTESIAN_POINT('Ctrl Pts',(3.15028249772165,-8.17819102774086,107.810691841183));
#47875=CARTESIAN_POINT('Ctrl Pts',(3.45014823017616,-8.19795880172907,108.136232436432));
#47876=CARTESIAN_POINT('Ctrl Pts',(3.34096054396247,-8.2177265757173,108.565154557429));
#47877=CARTESIAN_POINT('Ctrl Pts',(2.92193919249646,-8.23749434970552,108.707693126379));
#47878=CARTESIAN_POINT('Ctrl Pts',(2.57385234217612,-8.25726212369374,108.434322167266));
#47879=CARTESIAN_POINT('Ctrl Pts',(2.61300939186774,-8.27702989768196,107.993456130795));
#47880=CARTESIAN_POINT('Ctrl Pts',(3.00382800675135,-8.29679767167018,107.785713629347));
#47881=CARTESIAN_POINT('Ctrl Pts',(3.3911680802534,-8.3165654456584,107.99987199157));
#47882=CARTESIAN_POINT('Ctrl Pts',(3.42305048510065,-8.33633321964662,108.44132374308));
#47883=CARTESIAN_POINT('Ctrl Pts',(3.07050341641071,-8.35610099363484,108.708918027413));
#47884=CARTESIAN_POINT('Ctrl Pts',(2.65388931031493,-8.37586876762306,108.559489705961));
#47885=CARTESIAN_POINT('Ctrl Pts',(2.55178884953464,-8.39563654161128,108.128825529881));
#47886=CARTESIAN_POINT('Ctrl Pts',(2.85698156693412,-8.4154043155995,107.808273596653));
#47887=CARTESIAN_POINT('Ctrl Pts',(3.29213631691856,-8.43517208958772,107.889122098284));
#47888=CARTESIAN_POINT('Ctrl Pts',(3.4618243803737,-8.45493986357594,108.297903332895));
#47889=CARTESIAN_POINT('Ctrl Pts',(3.21184881107887,-8.47470763756417,108.663154412846));
#47890=CARTESIAN_POINT('Ctrl Pts',(2.76936447561803,-8.49447541155238,108.652968661937));
#47891=CARTESIAN_POINT('Ctrl Pts',(2.53646054802784,-8.51424318554061,108.276601956232));
#47892=CARTESIAN_POINT('Ctrl Pts',(2.72477875292914,-8.53401095952883,107.876061832958));
#47893=CARTESIAN_POINT('Ctrl Pts',(3.16319278053749,-8.55377873351705,107.815322413747));
#47894=CARTESIAN_POINT('Ctrl Pts',(3.45331217921457,-8.57354650750527,108.149578111023));
#47895=CARTESIAN_POINT('Ctrl Pts',(3.33150305271275,-8.59331428149349,108.575088009087));
#47896=CARTESIAN_POINT('Ctrl Pts',(2.90845436138638,-8.61308205548171,108.705187745508));
#47897=CARTESIAN_POINT('Ctrl Pts',(2.56859394875574,-8.63284982946993,108.421654614153));
#47898=CARTESIAN_POINT('Ctrl Pts',(2.62075578170033,-8.65261760345815,107.982137515698));
#47899=CARTESIAN_POINT('Ctrl Pts',(3.0175399713561,-8.67238537744638,107.786029271381));
#47900=CARTESIAN_POINT('Ctrl Pts',(3.39838544402236,-8.6921531514346,108.01153506421));
#47901=CARTESIAN_POINT('Ctrl Pts',(3.41721476990605,-8.71192092542281,108.453735915789));
#47902=CARTESIAN_POINT('Ctrl Pts',(3.05691758489821,-8.73168869941104,108.710800256228));
#47903=CARTESIAN_POINT('Ctrl Pts',(2.64489891990612,-8.75145647339926,108.549131593995));
#47904=CARTESIAN_POINT('Ctrl Pts',(2.55556354232526,-8.77122424738748,108.115639579118));
#47905=CARTESIAN_POINT('Ctrl Pts',(2.87009124837673,-8.7909920213757,107.804241989571));
#47906=CARTESIAN_POINT('Ctrl Pts',(3.30266811109706,-8.81075979536392,107.89790838957));
#47907=CARTESIAN_POINT('Ctrl Pts',(3.4602079588426,-8.83052756935214,108.311523347015));
#47908=CARTESIAN_POINT('Ctrl Pts',(3.19955302944784,-8.85029534334036,108.66923153036));
#47909=CARTESIAN_POINT('Ctrl Pts',(2.75756261231512,-8.87006311732858,108.645980555915));
#47910=CARTESIAN_POINT('Ctrl Pts',(2.5358770538127,-8.8898308913168,108.262898776393));
#47911=CARTESIAN_POINT('Ctrl Pts',(2.73594385381932,-8.90959866530503,107.868095772118));
#47912=CARTESIAN_POINT('Ctrl Pts',(3.17596065704247,-8.92936643929324,107.820332297254));
#47913=CARTESIAN_POINT('Ctrl Pts',(3.45608055639113,-8.94913421328146,108.163011416312));
#47914=CARTESIAN_POINT('Ctrl Pts',(3.32175628333195,-8.96890198726969,108.584737780578));
#47915=CARTESIAN_POINT('Ctrl Pts',(2.89504941536962,-8.9886697612579,108.702285156064));
#47916=CARTESIAN_POINT('Ctrl Pts',(2.56371201137874,-9.00843753524613,108.408837270799));
#47917=CARTESIAN_POINT('Ctrl Pts',(2.62883310982096,-9.02820530923435,107.971052644313));
#47918=CARTESIAN_POINT('Ctrl Pts',(3.0312366301285,-9.04797308322257,107.786749786241));
#47919=CARTESIAN_POINT('Ctrl Pts',(3.40525516637858,-9.06774085721079,108.023406227504));
#47920=CARTESIAN_POINT('Ctrl Pts',(3.41101498234141,-9.08750863119901,108.465970303283));
#47921=CARTESIAN_POINT('Ctrl Pts',(3.04328208563524,-9.10727640518723,108.712280378853));
#47922=CARTESIAN_POINT('Ctrl Pts',(2.63621839985404,-9.12704417917545,108.538512452087));
#47923=CARTESIAN_POINT('Ctrl Pts',(2.55972606184133,-9.14681195316367,108.10257087472));
#47924=CARTESIAN_POINT('Ctrl Pts',(2.88331429152557,-9.16657972715189,107.800599362433));
#47925=CARTESIAN_POINT('Ctrl Pts',(3.31293578932116,-9.18634750114011,107.907001925059));
#47926=CARTESIAN_POINT('Ctrl Pts',(3.45818994787757,-9.20611527512833,108.325089674315));
#47927=CARTESIAN_POINT('Ctrl Pts',(3.18708311291289,-9.22588304911656,108.674942815543));
#47928=CARTESIAN_POINT('Ctrl Pts',(2.7459723056586,-9.24565082310477,108.638646907232));
#47929=CARTESIAN_POINT('Ctrl Pts',(2.53569856627601,-9.265418597093,108.249184340345));
#47930=CARTESIAN_POINT('Ctrl Pts',(2.74733937468242,-9.28518637108122,107.860462971636));
#47931=CARTESIAN_POINT('Ctrl Pts',(3.1885749905948,-9.30495414506944,107.825717117965));
#47932=CARTESIAN_POINT('Ctrl Pts',(3.45845093534624,-9.32472191905766,108.176520634247));
#47933=CARTESIAN_POINT('Ctrl Pts',(3.31172876411578,-9.34448969304588,108.59409544218));
#47934=CARTESIAN_POINT('Ctrl Pts',(2.88173600190796,-9.3642574670341,108.698987910636));
#47935=CARTESIAN_POINT('Ctrl Pts',(2.55921089908849,-9.38402524102233,108.395881278955));
#47936=CARTESIAN_POINT('Ctrl Pts',(2.63723409084994,-9.40379301501054,107.960211282797));
#47937=CARTESIAN_POINT('Ctrl Pts',(3.04490654720541,-9.42356078899876,107.787874341084));
#47938=CARTESIAN_POINT('Ctrl Pts',(3.41177013152627,-9.44332856298698,108.035475562137));
#47939=CARTESIAN_POINT('Ctrl Pts',(3.40445898046695,-9.46309633697521,108.478015256788));
#47940=CARTESIAN_POINT('Ctrl Pts',(3.02960351867329,-9.48286411096342,108.713359165034));
#47941=CARTESIAN_POINT('Ctrl Pts',(2.62786695879146,-9.50263188495165,108.5276368633));
#47942=CARTESIAN_POINT('Ctrl Pts',(2.564247820732,-9.52239965893987,108.089640312703));
#47943=CARTESIAN_POINT('Ctrl Pts',(2.89669475751776,-9.54216743292808,107.797325749426));
#47944=CARTESIAN_POINT('Ctrl Pts',(3.32281396453211,-9.56193520691631,107.916436313859));
#47945=CARTESIAN_POINT('Ctrl Pts',(3.45604186940558,-9.58170298090453,108.33846864974));
#47946=CARTESIAN_POINT('Ctrl Pts',(3.17391765693164,-9.60147075489275,108.680439006897));
#47947=CARTESIAN_POINT('Ctrl Pts',(2.80901503514533,-9.61794389988293,108.638571606125));
#47948=CARTESIAN_POINT('Ctrl Pts',(2.63400072406848,-9.63112241587508,108.433469413069));
#47949=CARTESIAN_POINT('Ctrl Pts',(2.60485441639831,-9.63771167387116,108.302793470514));
#47950=CARTESIAN_POINT('Ctrl Pts',(2.60689261640396,-9.64100630286919,108.237692483505));
#47951=CARTESIAN_POINT('',(3.1742900872407,-9.6,108.602573191677));
#47952=CARTESIAN_POINT('Ctrl Pts',(3.17429377121672,-9.6,108.603153754506));
#47953=CARTESIAN_POINT('Ctrl Pts',(3.16531402749991,-9.6,108.606703341212));
#47954=CARTESIAN_POINT('Ctrl Pts',(3.15621182021442,-9.6,108.609893144108));
#47955=CARTESIAN_POINT('Ctrl Pts',(3.14699950494929,-9.6,108.612705889));
#47956=CARTESIAN_POINT('Ctrl Pts',(3.13221297128382,-9.6,108.617220578938));
#47957=CARTESIAN_POINT('Ctrl Pts',(3.11714267480703,-9.6,108.620764531874));
#47958=CARTESIAN_POINT('Ctrl Pts',(3.10187550064643,-9.6,108.623357279418));
#47959=CARTESIAN_POINT('Ctrl Pts',(3.09495631027381,-9.6,108.624532330784));
#47960=CARTESIAN_POINT('Ctrl Pts',(3.08799668415841,-9.6,108.625511820671));
#47961=CARTESIAN_POINT('Ctrl Pts',(3.08100483727106,-9.6,108.626296670564));
#47962=CARTESIAN_POINT('Ctrl Pts',(3.07531757538958,-9.6,108.626935077976));
#47963=CARTESIAN_POINT('Ctrl Pts',(3.06961045465332,-9.6,108.627444386443));
#47964=CARTESIAN_POINT('Ctrl Pts',(3.06389748778519,-9.6,108.627824830137));
#47965=CARTESIAN_POINT('Ctrl Pts',(3.04242911949262,-9.6,108.629254473532));
#47966=CARTESIAN_POINT('Ctrl Pts',(3.02083984010078,-9.6,108.628872863495));
#47967=CARTESIAN_POINT('Ctrl Pts',(2.9993685461102,-9.6,108.626720448274));
#47968=CARTESIAN_POINT('Ctrl Pts',(2.99279738093697,-9.6,108.626061714061));
#47969=CARTESIAN_POINT('Ctrl Pts',(2.98623737278602,-9.6,108.625236767709));
#47970=CARTESIAN_POINT('Ctrl Pts',(2.97969575955364,-9.6,108.624245868345));
#47971=CARTESIAN_POINT('Ctrl Pts',(2.9737973953897,-9.6,108.62335240597));
#47972=CARTESIAN_POINT('Ctrl Pts',(2.96792150025955,-9.6,108.62232506083));
#47973=CARTESIAN_POINT('Ctrl Pts',(2.96207934152988,-9.6,108.621166234703));
#47974=CARTESIAN_POINT('Ctrl Pts',(2.94154727022957,-9.6,108.61709357907));
#47975=CARTESIAN_POINT('Ctrl Pts',(2.9214053619483,-9.6,108.611396770555));
#47976=CARTESIAN_POINT('Ctrl Pts',(2.90187585569679,-9.6,108.604107979702));
#47977=CARTESIAN_POINT('Ctrl Pts',(2.88931665049007,-9.6,108.599420640511));
#47978=CARTESIAN_POINT('Ctrl Pts',(2.87701101845743,-9.6,108.594073939369));
#47979=CARTESIAN_POINT('Ctrl Pts',(2.86502492333012,-9.6,108.588067088395));
#47980=CARTESIAN_POINT('Ctrl Pts',(2.85938306415935,-9.6,108.58523966154));
#47981=CARTESIAN_POINT('Ctrl Pts',(2.85381209862818,-9.6,108.582265874473));
#47982=CARTESIAN_POINT('Ctrl Pts',(2.84831949871591,-9.6,108.579145145521));
#47983=CARTESIAN_POINT('Ctrl Pts',(2.84383384959628,-9.6,108.576596535518));
#47984=CARTESIAN_POINT('Ctrl Pts',(2.83940054726157,-9.6,108.573949716596));
#47985=CARTESIAN_POINT('Ctrl Pts',(2.83503573984888,-9.6,108.571212399444));
#47986=CARTESIAN_POINT('Ctrl Pts',(2.82136363059275,-9.6,108.562638161079));
#47987=CARTESIAN_POINT('Ctrl Pts',(2.80833101955341,-9.6,108.553159962205));
#47988=CARTESIAN_POINT('Ctrl Pts',(2.79604816320949,-9.6,108.542784903682));
#47989=CARTESIAN_POINT('Ctrl Pts',(2.78292483917589,-9.6,108.531699920591));
#47990=CARTESIAN_POINT('Ctrl Pts',(2.77065685708771,-9.6,108.519590661791));
#47991=CARTESIAN_POINT('Ctrl Pts',(2.75932851942847,-9.6,108.506587814261));
#47992=CARTESIAN_POINT('Ctrl Pts',(2.75483050724524,-9.6,108.501424923786));
#47993=CARTESIAN_POINT('Ctrl Pts',(2.75048091227549,-9.6,108.496121027901));
#47994=CARTESIAN_POINT('Ctrl Pts',(2.7462861731423,-9.6,108.490683960116));
#47995=CARTESIAN_POINT('Ctrl Pts',(2.74283580266206,-9.6,108.486211715815));
#47996=CARTESIAN_POINT('Ctrl Pts',(2.73948942853888,-9.6,108.481647829372));
#47997=CARTESIAN_POINT('Ctrl Pts',(2.73626148259601,-9.6,108.477012896759));
#47998=CARTESIAN_POINT('Ctrl Pts',(2.72501814129942,-9.6,108.460868844106));
#47999=CARTESIAN_POINT('Ctrl Pts',(2.715174764228,-9.6,108.443823493711));
#48000=CARTESIAN_POINT('Ctrl Pts',(2.70685061558342,-9.6,108.426080197397));
#48001=CARTESIAN_POINT('Ctrl Pts',(2.70318585754897,-9.6,108.41826860122));
#48002=CARTESIAN_POINT('Ctrl Pts',(2.69981619459356,-9.6,108.4103214895));
#48003=CARTESIAN_POINT('Ctrl Pts',(2.69675497973943,-9.6,108.40225562313));
#48004=CARTESIAN_POINT('Ctrl Pts',(2.69257854818296,-9.6,108.391251319139));
#48005=CARTESIAN_POINT('Ctrl Pts',(2.68897600041125,-9.6,108.380025872053));
#48006=CARTESIAN_POINT('Ctrl Pts',(2.68596529828858,-9.6,108.368622420101));
#48007=CARTESIAN_POINT('Ctrl Pts',(2.6847911110125,-9.6,108.364175022902));
#48008=CARTESIAN_POINT('Ctrl Pts',(2.68370798559853,-9.6,108.359703786269));
#48009=CARTESIAN_POINT('Ctrl Pts',(2.68271831874412,-9.6,108.355219601019));
#48010=CARTESIAN_POINT('Ctrl Pts',(2.67853974726888,-9.6,108.336286473683));
#48011=CARTESIAN_POINT('Ctrl Pts',(2.67601119798638,-9.6,108.317078942186));
#48012=CARTESIAN_POINT('Ctrl Pts',(2.6751801965963,-9.6,108.297794014685));
#48013=CARTESIAN_POINT('Ctrl Pts',(2.67434919520622,-9.6,108.278509087184));
#48014=CARTESIAN_POINT('Ctrl Pts',(2.67521572840128,-9.6,108.259145218824));
#48015=CARTESIAN_POINT('Ctrl Pts',(2.67788283232033,-9.6,108.239915065145));
#48016=CARTESIAN_POINT('Ctrl Pts',(2.60706672186757,-9.51538364779651,108.249732606859));
#48017=CARTESIAN_POINT('Ctrl Pts',(2.60676993033995,-9.51772231817763,108.203380299727));
#48018=CARTESIAN_POINT('Ctrl Pts',(2.61435669847727,-9.52006098855875,108.157121182639));
#48019=CARTESIAN_POINT('Ctrl Pts',(2.6302588332062,-9.52239965893987,108.113920643923));
#48020=CARTESIAN_POINT('Ctrl Pts',(2.67506346632725,-9.52898891693594,107.992202124944));
#48021=CARTESIAN_POINT('Ctrl Pts',(2.7858791119225,-9.53557817493201,107.894763937185));
#48022=CARTESIAN_POINT('Ctrl Pts',(2.91230680255585,-9.54216743292809,107.865896604045));
#48023=CARTESIAN_POINT('Ctrl Pts',(3.03873449318921,-9.54875669092416,107.837029270904));
#48024=CARTESIAN_POINT('Ctrl Pts',(3.18077422886066,-9.55534594892024,107.876732792381));
#48025=CARTESIAN_POINT('Ctrl Pts',(3.27399874750863,-9.56193520691631,107.966923275767));
#48026=CARTESIAN_POINT('Ctrl Pts',(3.3672232661566,-9.56852446491238,108.057113759153));
#48027=CARTESIAN_POINT('Ctrl Pts',(3.41163256778109,-9.57511372290845,108.197791204446));
#48028=CARTESIAN_POINT('Ctrl Pts',(3.38681651651434,-9.58170298090453,108.325124986619));
#48029=CARTESIAN_POINT('Ctrl Pts',(3.36384682027175,-9.58780198726969,108.442984925999));
#48030=CARTESIAN_POINT('Ctrl Pts',(3.2815695271407,-9.59390099363484,108.549412917973));
#48031=CARTESIAN_POINT('Ctrl Pts',(3.17429377121673,-9.6,108.603153754506));
#48032=CARTESIAN_POINT('',(2.81284134682606,-7.7433,107.987639915065));
#48033=CARTESIAN_POINT('Ctrl Pts',(2.81242348876314,-7.7433,107.987412508431));
#48034=CARTESIAN_POINT('Ctrl Pts',(2.80543771171585,-7.7433,107.991294650159));
#48035=CARTESIAN_POINT('Ctrl Pts',(2.79862088669944,-7.7433,107.995444194259));
#48036=CARTESIAN_POINT('Ctrl Pts',(2.79199078672996,-7.7433,107.999857486819));
#48037=CARTESIAN_POINT('Ctrl Pts',(2.77908729716369,-7.7433,108.008446629481));
#48038=CARTESIAN_POINT('Ctrl Pts',(2.76689025213856,-7.7433,108.018033178706));
#48039=CARTESIAN_POINT('Ctrl Pts',(2.75543032796706,-7.7433,108.028491416979));
#48040=CARTESIAN_POINT('Ctrl Pts',(2.74885145575796,-7.7433,108.034495244937));
#48041=CARTESIAN_POINT('Ctrl Pts',(2.74251154039275,-7.7433,108.040791956438));
#48042=CARTESIAN_POINT('Ctrl Pts',(2.73644185997739,-7.7433,108.047333637481));
#48043=CARTESIAN_POINT('Ctrl Pts',(2.72536667462749,-7.7433,108.059270069895));
#48044=CARTESIAN_POINT('Ctrl Pts',(2.71517634671577,-7.7433,108.072031116775));
#48045=CARTESIAN_POINT('Ctrl Pts',(2.70590800409384,-7.7433,108.085481282292));
#48046=CARTESIAN_POINT('Ctrl Pts',(2.70149813712292,-7.7433,108.091880855883));
#48047=CARTESIAN_POINT('Ctrl Pts',(2.69729719824473,-7.7433,108.098436790851));
#48048=CARTESIAN_POINT('Ctrl Pts',(2.69331048318176,-7.7433,108.105136166992));
#48049=CARTESIAN_POINT('Ctrl Pts',(2.69029373455844,-7.7433,108.110205587161));
#48050=CARTESIAN_POINT('Ctrl Pts',(2.68740348024832,-7.7433,108.115350995326));
#48051=CARTESIAN_POINT('Ctrl Pts',(2.68464466603131,-7.7433,108.120559727848));
#48052=CARTESIAN_POINT('Ctrl Pts',(2.67526428768186,-7.7433,108.138270192538));
#48053=CARTESIAN_POINT('Ctrl Pts',(2.66738748661794,-7.7433,108.156731872377));
#48054=CARTESIAN_POINT('Ctrl Pts',(2.66108511861829,-7.7433,108.175717308618));
#48055=CARTESIAN_POINT('Ctrl Pts',(2.65701462694751,-7.7433,108.187979375843));
#48056=CARTESIAN_POINT('Ctrl Pts',(2.65360153253527,-7.7433,108.200460875424));
#48057=CARTESIAN_POINT('Ctrl Pts',(2.65087412228317,-7.7433,108.213107378602));
#48058=CARTESIAN_POINT('Ctrl Pts',(2.64967297503825,-7.7433,108.218676878987));
#48059=CARTESIAN_POINT('Ctrl Pts',(2.64860492320512,-7.7433,108.224278432823));
#48060=CARTESIAN_POINT('Ctrl Pts',(2.64767292173802,-7.7433,108.229907575979));
#48061=CARTESIAN_POINT('Ctrl Pts',(2.64685670237713,-7.7433,108.234837413315));
#48062=CARTESIAN_POINT('Ctrl Pts',(2.64614551927426,-7.7433,108.239785185843));
#48063=CARTESIAN_POINT('Ctrl Pts',(2.64554197116888,-7.7433,108.244737602616));
#48064=CARTESIAN_POINT('Ctrl Pts',(2.64363794439926,-7.7433,108.26036110309));
#48065=CARTESIAN_POINT('Ctrl Pts',(2.64279904357055,-7.7433,108.276058873989));
#48066=CARTESIAN_POINT('Ctrl Pts',(2.64306324300403,-7.7433,108.291731172273));
#48067=CARTESIAN_POINT('Ctrl Pts',(2.64332016877862,-7.7433,108.306971997444));
#48068=CARTESIAN_POINT('Ctrl Pts',(2.64462004986702,-7.7433,108.322189111009));
#48069=CARTESIAN_POINT('Ctrl Pts',(2.64690694953374,-7.7433,108.337294815271));
#48070=CARTESIAN_POINT('Ctrl Pts',(2.64820783454331,-7.7433,108.34588757713));
#48071=CARTESIAN_POINT('Ctrl Pts',(2.64982842986809,-7.7433,108.354444353112));
#48072=CARTESIAN_POINT('Ctrl Pts',(2.65176092930574,-7.7433,108.3629490723));
#48073=CARTESIAN_POINT('Ctrl Pts',(2.65319972813317,-7.7433,108.369281068965));
#48074=CARTESIAN_POINT('Ctrl Pts',(2.6548126015421,-7.7433,108.375587189865));
#48075=CARTESIAN_POINT('Ctrl Pts',(2.65658913504752,-7.7433,108.381836343915));
#48076=CARTESIAN_POINT('Ctrl Pts',(2.66230148532117,-7.7433,108.401930170878));
#48077=CARTESIAN_POINT('Ctrl Pts',(2.66971154967432,-7.7433,108.421485690035));
#48078=CARTESIAN_POINT('Ctrl Pts',(2.6786763255829,-7.7433,108.4402892797));
#48079=CARTESIAN_POINT('Ctrl Pts',(2.68292788902861,-7.7433,108.449206920841));
#48080=CARTESIAN_POINT('Ctrl Pts',(2.68752991854632,-7.7433,108.457955507247));
#48081=CARTESIAN_POINT('Ctrl Pts',(2.69247119621592,-7.7433,108.466511877091));
#48082=CARTESIAN_POINT('Ctrl Pts',(2.69850572248428,-7.7433,108.47696132803));
#48083=CARTESIAN_POINT('Ctrl Pts',(2.70504610294034,-7.7433,108.487124226895));
#48084=CARTESIAN_POINT('Ctrl Pts',(2.71206752469552,-7.7433,108.496973445774));
#48085=CARTESIAN_POINT('Ctrl Pts',(2.71519702499412,-7.7433,108.501363316444));
#48086=CARTESIAN_POINT('Ctrl Pts',(2.71842256404046,-7.7433,108.505691035234));
#48087=CARTESIAN_POINT('Ctrl Pts',(2.72173214836912,-7.7433,108.50994201636));
#48088=CARTESIAN_POINT('Ctrl Pts',(2.73493899592972,-7.7433,108.526905493988));
#48089=CARTESIAN_POINT('Ctrl Pts',(2.74951416763527,-7.7433,108.542697494939));
#48090=CARTESIAN_POINT('Ctrl Pts',(2.7652868091383,-7.7433,108.557185273403));
#48091=CARTESIAN_POINT('Ctrl Pts',(2.78107258747146,-7.7433,108.57168511855));
#48092=CARTESIAN_POINT('Ctrl Pts',(2.79805862616208,-7.7433,108.584879730222));
#48093=CARTESIAN_POINT('Ctrl Pts',(2.81611663889779,-7.7433,108.596608595281));
#48094=CARTESIAN_POINT('Ctrl Pts',(2.81909225249591,-7.7433,108.598541286928));
#48095=CARTESIAN_POINT('Ctrl Pts',(2.82209705219277,-7.7433,108.600434096425));
#48096=CARTESIAN_POINT('Ctrl Pts',(2.82513055246694,-7.7433,108.602286199445));
#48097=CARTESIAN_POINT('Ctrl Pts',(2.81242348876314,-7.7433,107.987412508431));
#48098=CARTESIAN_POINT('Ctrl Pts',(2.89276360714258,-7.74939900636515,107.930741660299));
#48099=CARTESIAN_POINT('Ctrl Pts',(3.11892943575575,-7.76208727072639,107.892835510919));
#48100=CARTESIAN_POINT('Ctrl Pts',(3.36586763099966,-7.78136479308369,108.145991153067));
#48101=CARTESIAN_POINT('Ctrl Pts',(3.2869314131236,-7.80113256707191,108.499845495719));
#48102=CARTESIAN_POINT('Ctrl Pts',(2.9471249283031,-7.82090034106013,108.626779562835));
#48103=CARTESIAN_POINT('Ctrl Pts',(2.70982409425543,-7.83698193367859,108.451463078785));
#48104=CARTESIAN_POINT('Ctrl Pts',(2.67804342236209,-7.84647426830099,108.297299382674));
#48105=CARTESIAN_POINT('Ctrl Pts',(2.6781760831613,-7.84937734492731,108.250099030543));
#48106=CARTESIAN_POINT('Origin',(3.,-7.7433,108.25));
#48107=CARTESIAN_POINT('',(2.6067,-7.7433,108.25));
#48108=CARTESIAN_POINT('Origin',(3.,-7.7433,108.25));
#48109=CARTESIAN_POINT('Origin',(3.,-7.7433,108.25));
#48110=CARTESIAN_POINT('',(3.18715865317386,-7.7433,107.987639915065));
#48111=CARTESIAN_POINT('Ctrl Pts',(3.17532910733317,-7.7433,108.602640901019));
#48112=CARTESIAN_POINT('Ctrl Pts',(3.18359398155869,-7.7433,108.597648184601));
#48113=CARTESIAN_POINT('Ctrl Pts',(3.19164684676494,-7.7433,108.592340041651));
#48114=CARTESIAN_POINT('Ctrl Pts',(3.19946647439599,-7.7433,108.586715834233));
#48115=CARTESIAN_POINT('Ctrl Pts',(3.21201762835566,-7.7433,108.57768851266));
#48116=CARTESIAN_POINT('Ctrl Pts',(3.22396848685653,-7.7433,108.56784725185));
#48117=CARTESIAN_POINT('Ctrl Pts',(3.23528194102692,-7.7433,108.557273005132));
#48118=CARTESIAN_POINT('Ctrl Pts',(3.2404092782778,-7.7433,108.552480681914));
#48119=CARTESIAN_POINT('Ctrl Pts',(3.24540554458826,-7.7433,108.54753769427));
#48120=CARTESIAN_POINT('Ctrl Pts',(3.25026649528812,-7.7433,108.542451135696));
#48121=CARTESIAN_POINT('Ctrl Pts',(3.25422045744394,-7.7433,108.538313661086));
#48122=CARTESIAN_POINT('Ctrl Pts',(3.25808375246127,-7.7433,108.534082163145));
#48123=CARTESIAN_POINT('Ctrl Pts',(3.26184807585996,-7.7433,108.529767931107));
#48124=CARTESIAN_POINT('Ctrl Pts',(3.27599376874567,-7.7433,108.513555774238));
#48125=CARTESIAN_POINT('Ctrl Pts',(3.28877184484755,-7.7433,108.496149932804));
#48126=CARTESIAN_POINT('Ctrl Pts',(3.30006972609028,-7.7433,108.477764961624));
#48127=CARTESIAN_POINT('Ctrl Pts',(3.3035273783011,-7.7433,108.4721383459));
#48128=CARTESIAN_POINT('Ctrl Pts',(3.30684604562309,-7.7433,108.466419892314));
#48129=CARTESIAN_POINT('Ctrl Pts',(3.31002154851212,-7.7433,108.460615515744));
#48130=CARTESIAN_POINT('Ctrl Pts',(3.31288479673219,-7.7433,108.455381897177));
#48131=CARTESIAN_POINT('Ctrl Pts',(3.3156279244079,-7.7433,108.450085029156));
#48132=CARTESIAN_POINT('Ctrl Pts',(3.31824601493307,-7.7433,108.444735330345));
#48133=CARTESIAN_POINT('Ctrl Pts',(3.32744720835576,-7.7433,108.425933989045));
#48134=CARTESIAN_POINT('Ctrl Pts',(3.33511994980111,-7.7433,108.406458901024));
#48135=CARTESIAN_POINT('Ctrl Pts',(3.34115516947733,-7.7433,108.386506354067));
#48136=CARTESIAN_POINT('Ctrl Pts',(3.3450363511826,-7.7433,108.373675096155));
#48137=CARTESIAN_POINT('Ctrl Pts',(3.34823935165694,-7.7433,108.360646030631));
#48138=CARTESIAN_POINT('Ctrl Pts',(3.35072357452333,-7.7433,108.347471155269));
#48139=CARTESIAN_POINT('Ctrl Pts',(3.35189289819558,-7.7433,108.3412697416));
#48140=CARTESIAN_POINT('Ctrl Pts',(3.35290283345036,-7.7433,108.335036040526));
#48141=CARTESIAN_POINT('Ctrl Pts',(3.35374839004862,-7.7433,108.328775643654));
#48142=CARTESIAN_POINT('Ctrl Pts',(3.35443893300448,-7.7433,108.323662948691));
#48143=CARTESIAN_POINT('Ctrl Pts',(3.35501963039338,-7.7433,108.318532388353));
#48144=CARTESIAN_POINT('Ctrl Pts',(3.35548683149189,-7.7433,108.31340148095));
#48145=CARTESIAN_POINT('Ctrl Pts',(3.35695026851071,-7.7433,108.2973296869));
#48146=CARTESIAN_POINT('Ctrl Pts',(3.35730709707381,-7.7433,108.281218884331));
#48147=CARTESIAN_POINT('Ctrl Pts',(3.35649615794086,-7.7433,108.265161086695));
#48148=CARTESIAN_POINT('Ctrl Pts',(3.35562972897909,-7.7433,108.248004508144));
#48149=CARTESIAN_POINT('Ctrl Pts',(3.35343019058695,-7.7433,108.230907725327));
#48150=CARTESIAN_POINT('Ctrl Pts',(3.34995042508722,-7.7433,108.214016990077));
#48151=CARTESIAN_POINT('Ctrl Pts',(3.34856875501914,-7.7433,108.207310382024));
#48152=CARTESIAN_POINT('Ctrl Pts',(3.34698498184747,-7.7433,108.200636402444));
#48153=CARTESIAN_POINT('Ctrl Pts',(3.34520143590219,-7.7433,108.194004919961));
#48154=CARTESIAN_POINT('Ctrl Pts',(3.34373439173525,-7.7433,108.188550236991));
#48155=CARTESIAN_POINT('Ctrl Pts',(3.34213143104911,-7.7433,108.183122755611));
#48156=CARTESIAN_POINT('Ctrl Pts',(3.34040019349256,-7.7433,108.177746436119));
#48157=CARTESIAN_POINT('Ctrl Pts',(3.33437005187905,-7.7433,108.159019966273));
#48158=CARTESIAN_POINT('Ctrl Pts',(3.32677462929342,-7.7433,108.140861064214));
#48159=CARTESIAN_POINT('Ctrl Pts',(3.31770342973941,-7.7433,108.123487824168));
#48160=CARTESIAN_POINT('Ctrl Pts',(3.31370977647758,-7.7433,108.11583914481));
#48161=CARTESIAN_POINT('Ctrl Pts',(3.30942951053824,-7.7433,108.10834310507));
#48162=CARTESIAN_POINT('Ctrl Pts',(3.30486787449355,-7.7433,108.101020483498));
#48163=CARTESIAN_POINT('Ctrl Pts',(3.29864441319003,-7.7433,108.091030196779));
#48164=CARTESIAN_POINT('Ctrl Pts',(3.29189729436454,-7.7433,108.081362445845));
#48165=CARTESIAN_POINT('Ctrl Pts',(3.2846499513607,-7.7433,108.072057658498));
#48166=CARTESIAN_POINT('Ctrl Pts',(3.28182345518518,-7.7433,108.068428749829));
#48167=CARTESIAN_POINT('Ctrl Pts',(3.27892281702297,-7.7433,108.064857837219));
#48168=CARTESIAN_POINT('Ctrl Pts',(3.27595524844569,-7.7433,108.06135342638));
#48169=CARTESIAN_POINT('Ctrl Pts',(3.2634255806509,-7.7433,108.046557103233));
#48170=CARTESIAN_POINT('Ctrl Pts',(3.24967781791732,-7.7433,108.032907128281));
#48171=CARTESIAN_POINT('Ctrl Pts',(3.23483988540938,-7.7433,108.02056068259));
#48172=CARTESIAN_POINT('Ctrl Pts',(3.22000195290144,-7.7433,108.008214236899));
#48173=CARTESIAN_POINT('Ctrl Pts',(3.20407262972842,-7.7433,107.997170373806));
#48174=CARTESIAN_POINT('Ctrl Pts',(3.18715865317386,-7.7433,107.987639915065));
#48175=CARTESIAN_POINT('Origin',(3.,-7.7433,108.25));
#48176=CARTESIAN_POINT('Origin',(3.,-7.51222265507269,108.25));
#48177=CARTESIAN_POINT('Ctrl Pts',(3.18715865317386,-7.7433,107.987639915065));
#48178=CARTESIAN_POINT('Ctrl Pts',(3.23060708786083,-7.74659462899803,108.018634532712));
#48179=CARTESIAN_POINT('Ctrl Pts',(3.30131753225317,-7.75318388699411,108.102515506643));
#48180=CARTESIAN_POINT('Ctrl Pts',(3.34811842236999,-7.76636240298626,108.318434681996));
#48181=CARTESIAN_POINT('Ctrl Pts',(3.19423247158511,-7.78283554797644,108.577086075122));
#48182=CARTESIAN_POINT('Ctrl Pts',(2.83123989782698,-7.80260332196466,108.591198967572));
#48183=CARTESIAN_POINT('Ctrl Pts',(2.683650632963,-7.81656569099675,108.381854103748));
#48184=CARTESIAN_POINT('Ctrl Pts',(2.67726567995051,-7.82393880203276,108.262849788895));
#48185=CARTESIAN_POINT('Ctrl Pts',(2.67736158403691,-7.82472265507269,108.25018840343));
#48186=CARTESIAN_POINT('Ctrl Pts',(3.22840585926081,-7.7022936971308,107.929819342472));
#48187=CARTESIAN_POINT('Ctrl Pts',(3.2814297344059,-7.70558832612884,107.967644749719));
#48188=CARTESIAN_POINT('Ctrl Pts',(3.36772379314303,-7.71217758412492,108.07001194248));
#48189=CARTESIAN_POINT('Ctrl Pts',(3.42483895901983,-7.72535610011706,108.33351674945));
#48190=CARTESIAN_POINT('Ctrl Pts',(3.23703865045203,-7.74182924510725,108.649171370244));
#48191=CARTESIAN_POINT('Ctrl Pts',(2.79404748061548,-7.76159701909547,108.666394551069));
#48192=CARTESIAN_POINT('Ctrl Pts',(2.53904127250649,-7.78136479308369,108.304686401361));
#48193=CARTESIAN_POINT('Ctrl Pts',(2.70248654639492,-7.8011325670719,107.893528865296));
#48194=CARTESIAN_POINT('Ctrl Pts',(3.1364678991552,-7.82090034106013,107.806185082179));
#48195=CARTESIAN_POINT('Ctrl Pts',(3.44635212159991,-7.84066811504835,108.122191599049));
#48196=CARTESIAN_POINT('Ctrl Pts',(3.35067176640996,-7.86043588903657,108.554314595457));
#48197=CARTESIAN_POINT('Ctrl Pts',(2.93631475070566,-7.88020366302479,108.709915415827));
#48198=CARTESIAN_POINT('Ctrl Pts',(2.57983739147979,-7.89997143701301,108.447582221347));
#48199=CARTESIAN_POINT('Ctrl Pts',(2.60516141258424,-7.91973921100123,108.005706756459));
#48200=CARTESIAN_POINT('Ctrl Pts',(2.98928028820116,-7.93950698498946,107.785821511096));
#48201=CARTESIAN_POINT('Ctrl Pts',(3.38313944150234,-7.95927475897767,107.987739588043));
#48202=CARTESIAN_POINT('Ctrl Pts',(3.42883698967919,-7.97904253296589,108.427975643658));
#48203=CARTESIAN_POINT('Ctrl Pts',(3.08484664817965,-7.99881030695412,108.706483864232));
#48204=CARTESIAN_POINT('Ctrl Pts',(2.66375553478411,-8.01857808094234,108.570181375511));
#48205=CARTESIAN_POINT('Ctrl Pts',(2.54821251073349,-8.03834585493055,108.142927445569));
#48206=CARTESIAN_POINT('Ctrl Pts',(2.84321253014143,-8.05811362891878,107.812971221026));
#48207=CARTESIAN_POINT('Ctrl Pts',(3.28068661206076,-8.077881402907,107.880146665863));
#48208=CARTESIAN_POINT('Ctrl Pts',(3.46309845243368,-8.09764917689522,108.283410891203));
#48209=CARTESIAN_POINT('Ctrl Pts',(3.22468889862713,-8.11741695088343,108.656314364447));
#48210=CARTESIAN_POINT('Ctrl Pts',(2.78210268568124,-8.13718472487166,108.659996614914));
#48211=CARTESIAN_POINT('Ctrl Pts',(2.53752156346275,-8.15695249885988,108.291111551816));
#48212=CARTESIAN_POINT('Ctrl Pts',(2.71319842039437,-8.1767202728481,107.884868081583));
#48213=CARTESIAN_POINT('Ctrl Pts',(3.1494942438801,-8.19648804683632,107.810423004522));
#48214=CARTESIAN_POINT('Ctrl Pts',(3.44994341198594,-8.21625582082455,108.135425177598));
#48215=CARTESIAN_POINT('Ctrl Pts',(3.34152528153087,-8.23602359481276,108.56454243909));
#48216=CARTESIAN_POINT('Ctrl Pts',(2.92276030406872,-8.25579136880098,108.70783238558));
#48217=CARTESIAN_POINT('Ctrl Pts',(2.57418367690396,-8.27555914278921,108.435086257996));
#48218=CARTESIAN_POINT('Ctrl Pts',(2.61254986313247,-8.29532691677743,107.994150717502));
#48219=CARTESIAN_POINT('Ctrl Pts',(3.00299519211957,-8.31509469076565,107.785707535342));
#48220=CARTESIAN_POINT('Ctrl Pts',(3.39071876526407,-8.33486246475387,107.999170754528));
#48221=CARTESIAN_POINT('Ctrl Pts',(3.42339296600063,-8.35463023874209,108.440564582897));
#48222=CARTESIAN_POINT('Ctrl Pts',(3.07132647797405,-8.37439801273031,108.708790799225));
#48223=CARTESIAN_POINT('Ctrl Pts',(2.65444502969431,-8.39416578671854,108.560110023074));
#48224=CARTESIAN_POINT('Ctrl Pts',(2.55157223993528,-8.41393356070675,108.129629705006));
#48225=CARTESIAN_POINT('Ctrl Pts',(2.85618946328992,-8.43370133469498,107.808530869205));
#48226=CARTESIAN_POINT('Ctrl Pts',(3.29148851035998,-8.45346910868319,107.888598682568));
#48227=CARTESIAN_POINT('Ctrl Pts',(3.46190953807653,-8.47323688267141,108.2970748611));
#48228=CARTESIAN_POINT('Ctrl Pts',(3.21258954953447,-8.49300465665963,108.662773724142));
#48229=CARTESIAN_POINT('Ctrl Pts',(2.77008767966747,-8.51277243064786,108.653381691296));
#48230=CARTESIAN_POINT('Ctrl Pts',(2.53650903617205,-8.53254020463608,108.277433380461));
#48231=CARTESIAN_POINT('Ctrl Pts',(2.72410846359058,-8.5523079786243,107.876556129986));
#48232=CARTESIAN_POINT('Ctrl Pts',(3.16241281117998,-8.57207575261252,107.815030411778));
#48233=CARTESIAN_POINT('Ctrl Pts',(3.45313129444197,-8.59184352660074,108.14876515466));
#48234=CARTESIAN_POINT('Ctrl Pts',(3.33208562401345,-8.61161130058896,108.574492838499));
#48235=CARTESIAN_POINT('Ctrl Pts',(2.90927100140282,-8.63137907457718,108.705351197129));
#48236=CARTESIAN_POINT('Ctrl Pts',(2.5689025699531,-8.6511468485654,108.422428158143));
#48237=CARTESIAN_POINT('Ctrl Pts',(2.62027593744494,-8.67091462255362,107.982818226238));
#48238=CARTESIAN_POINT('Ctrl Pts',(3.01670770009012,-8.69068239654185,107.785998581175));
#48239=CARTESIAN_POINT('Ctrl Pts',(3.39795703752631,-8.71045017053006,108.010820861702));
#48240=CARTESIAN_POINT('Ctrl Pts',(3.41757952470489,-8.73021794451828,108.452987202702));
#48241=CARTESIAN_POINT('Ctrl Pts',(3.0577440452905,-8.74998571850651,108.710697394335));
#48242=CARTESIAN_POINT('Ctrl Pts',(2.64543607450032,-8.76975349249472,108.549768054749));
#48243=CARTESIAN_POINT('Ctrl Pts',(2.55532327430049,-8.78952126648295,108.116437005369));
#48244=CARTESIAN_POINT('Ctrl Pts',(2.86929189127361,-8.80928904047117,107.804475753492));
#48245=CARTESIAN_POINT('Ctrl Pts',(3.30203604732418,-8.82905681445939,107.897366067954));
#48246=CARTESIAN_POINT('Ctrl Pts',(3.4603175499762,-8.84882458844761,108.310697751998));
#48247=CARTESIAN_POINT('Ctrl Pts',(3.20030468911872,-8.86859236243583,108.668872886961));
#48248=CARTESIAN_POINT('Ctrl Pts',(2.75827330116574,-8.88836013642405,108.646414766355));
#48249=CARTESIAN_POINT('Ctrl Pts',(2.5359009630086,-8.90812791041227,108.263731270057));
#48250=CARTESIAN_POINT('Ctrl Pts',(2.73525925687653,-8.92789568440049,107.868570055129));
#48251=CARTESIAN_POINT('Ctrl Pts',(3.17518965286302,-8.94766345838871,107.82001738472));
#48252=CARTESIAN_POINT('Ctrl Pts',(3.45592376284752,-8.96743123237694,108.162193471856));
#48253=CARTESIAN_POINT('Ctrl Pts',(3.32235618001346,-8.98719900636516,108.58416007709));
#48254=CARTESIAN_POINT('Ctrl Pts',(2.89586087120222,-9.00696678035337,108.70247265748));
#48255=CARTESIAN_POINT('Ctrl Pts',(2.56399764973763,-9.0267345543416,108.409619593032));
#48256=CARTESIAN_POINT('Ctrl Pts',(2.62833336876932,-9.04650232832981,107.971718884682));
#48257=CARTESIAN_POINT('Ctrl Pts',(3.03040562848843,-9.06627010231804,107.786694526614));
#48258=CARTESIAN_POINT('Ctrl Pts',(3.40484804221826,-9.08603787630626,108.02267968276));
#48259=CARTESIAN_POINT('Ctrl Pts',(3.41140169273562,-9.10580565029448,108.465232690641));
#48260=CARTESIAN_POINT('Ctrl Pts',(3.04411122368577,-9.1255734242827,108.712201973012));
#48261=CARTESIAN_POINT('Ctrl Pts',(2.63673652088457,-9.14534119827093,108.539164501099));
#48262=CARTESIAN_POINT('Ctrl Pts',(2.55946234514999,-9.16510897225914,108.103360856223));
#48263=CARTESIAN_POINT('Ctrl Pts',(2.88250837829689,-9.18487674624736,107.800809413777));
#48264=CARTESIAN_POINT('Ctrl Pts',(3.31232002033802,-9.20464452023558,107.906441170695));
#48265=CARTESIAN_POINT('Ctrl Pts',(3.45832387583295,-9.22441229422381,108.324267676709));
#48266=CARTESIAN_POINT('Ctrl Pts',(3.18784504000744,-9.24418006821202,108.674606529979));
#48267=CARTESIAN_POINT('Ctrl Pts',(2.74666985451794,-9.26394784220025,108.639101920787));
#48268=CARTESIAN_POINT('Ctrl Pts',(2.53569788572799,-9.28371561618846,108.250017174951));
#48269=CARTESIAN_POINT('Ctrl Pts',(2.74664104561622,-9.30348339017669,107.860916831198));
#48270=CARTESIAN_POINT('Ctrl Pts',(3.18781367206768,-9.32325116416491,107.825379560034));
#48271=CARTESIAN_POINT('Ctrl Pts',(3.45831826603152,-9.34301893815313,108.175698436513));
#48272=CARTESIAN_POINT('Ctrl Pts',(3.31234568839827,-9.36278671214135,108.593535664409));
#48273=CARTESIAN_POINT('Ctrl Pts',(2.88254107342349,-9.38255448612957,108.699199398396));
#48274=CARTESIAN_POINT('Ctrl Pts',(2.55947437314993,-9.40232226011779,108.396671482843));
#48275=CARTESIAN_POINT('Ctrl Pts',(2.63671255465142,-9.42209003410602,107.960862951622));
#48276=CARTESIAN_POINT('Ctrl Pts',(3.04408258286891,-9.44185780809423,107.787793567058));
#48277=CARTESIAN_POINT('Ctrl Pts',(3.41137353694225,-9.46162558208245,108.034739653178));
#48278=CARTESIAN_POINT('Ctrl Pts',(3.40489100622148,-9.48139335607067,108.477284935403));
#48279=CARTESIAN_POINT('Ctrl Pts',(3.03038134687606,-9.50116113005889,108.713317276513));
#48280=CARTESIAN_POINT('Ctrl Pts',(2.62847550512648,-9.52092890404712,108.528286005137));
#48281=CARTESIAN_POINT('Ctrl Pts',(2.56370021112967,-9.54069667803534,108.090490261637));
#48282=CARTESIAN_POINT('Ctrl Pts',(2.8963776495683,-9.56046445202356,107.797465456433));
#48283=CARTESIAN_POINT('Ctrl Pts',(3.2500595337559,-9.57693759701374,107.89654078295));
#48284=CARTESIAN_POINT('Ctrl Pts',(3.3904177724541,-9.59011611300589,108.126750448904));
#48285=CARTESIAN_POINT('Ctrl Pts',(3.39852125534571,-9.59670537100196,108.26039191063));
#48286=CARTESIAN_POINT('Ctrl Pts',(3.38620837767256,-9.6,108.324350380063));
#48287=CARTESIAN_POINT('Ctrl Pts',(3.21465679056516,-7.71596246475387,107.949092866669));
#48288=CARTESIAN_POINT('Ctrl Pts',(3.26448885222421,-7.71925709375191,107.98464134405));
#48289=CARTESIAN_POINT('Ctrl Pts',(3.34558837284641,-7.72584635174798,108.080846463868));
#48290=CARTESIAN_POINT('Ctrl Pts',(3.39926544680322,-7.73902486774013,108.328489393632));
#48291=CARTESIAN_POINT('Ctrl Pts',(3.22276992416306,-7.75549801273031,108.625142938537));
#48292=CARTESIAN_POINT('Ctrl Pts',(2.80644495301932,-7.77526578671853,108.64132935657));
#48293=CARTESIAN_POINT('Ctrl Pts',(2.56678904233463,-7.79503356070675,108.301394510814));
#48294=CARTESIAN_POINT('Ctrl Pts',(2.72039560058791,-7.81480133469497,107.914986923049));
#48295=CARTESIAN_POINT('Ctrl Pts',(3.12825310761566,-7.83456910868319,107.832900867024));
#48296=CARTESIAN_POINT('Ctrl Pts',(3.41948360779651,-7.85433688267141,108.129885125346));
#48297=CARTESIAN_POINT('Ctrl Pts',(3.32956280615123,-7.87410465665963,108.53599614123));
#48298=CARTESIAN_POINT('Ctrl Pts',(2.94014833391706,-7.89387243064786,108.682230448957));
#48299=CARTESIAN_POINT('Ctrl Pts',(2.60512940713378,-7.91364020463607,108.435688605557));
#48300=CARTESIAN_POINT('Ctrl Pts',(2.62892902905276,-7.9334079786243,108.020412178633));
#48301=CARTESIAN_POINT('Ctrl Pts',(2.9899255696068,-7.95317575261252,107.813763096971));
#48302=CARTESIAN_POINT('Ctrl Pts',(3.36007606423926,-7.97294352660074,108.003526557921));
#48303=CARTESIAN_POINT('Ctrl Pts',(3.40302281289135,-7.99271130058896,108.417262261091));
#48304=CARTESIAN_POINT('Ctrl Pts',(3.0797392380712,-8.01247907457718,108.679005462285));
#48305=CARTESIAN_POINT('Ctrl Pts',(2.68399603240422,-8.0322468485654,108.550907808094));
#48306=CARTESIAN_POINT('Ctrl Pts',(2.57540821072938,-8.05201462255362,108.149372761425));
#48307=CARTESIAN_POINT('Ctrl Pts',(2.85265047407456,-8.07178239654184,107.839278508954));
#48308=CARTESIAN_POINT('Ctrl Pts',(3.26379046270775,-8.09155017053007,107.90241027554));
#48309=CARTESIAN_POINT('Ctrl Pts',(3.43522188019526,-8.11131794451828,108.28139969657));
#48310=CARTESIAN_POINT('Ctrl Pts',(3.21116357527346,-8.13108571850651,108.631855954637));
#48311=CARTESIAN_POINT('Ctrl Pts',(2.79521918432476,-8.15085349249472,108.635316549168));
#48312=CARTESIAN_POINT('Ctrl Pts',(2.5653608133611,-8.17062126648295,108.288636809916));
#48313=CARTESIAN_POINT('Ctrl Pts',(2.73046266498416,-8.19038904047117,107.906847481961));
#48314=CARTESIAN_POINT('Ctrl Pts',(3.14049532136837,-8.21015681445939,107.836883684329));
#48315=CARTESIAN_POINT('Ctrl Pts',(3.42285871765904,-8.22992458844761,108.142322098321));
#48316=CARTESIAN_POINT('Ctrl Pts',(3.32096690105733,-8.24969236243583,108.545608311845));
#48317=CARTESIAN_POINT('Ctrl Pts',(2.92740980775846,-8.26946013642405,108.680272808339));
#48318=CARTESIAN_POINT('Ctrl Pts',(2.5998160223128,-8.28922791041227,108.423944846458));
#48319=CARTESIAN_POINT('Ctrl Pts',(2.63587272606239,-8.30899568440049,108.009551764446));
#48320=CARTESIAN_POINT('Ctrl Pts',(3.00281489419577,-8.32876345838872,107.813655982077));
#48321=CARTESIAN_POINT('Ctrl Pts',(3.36719914470057,-8.34853123237693,108.014269616431));
#48322=CARTESIAN_POINT('Ctrl Pts',(3.39790649646067,-8.36829900636515,108.429093399322));
#48323=CARTESIAN_POINT('Ctrl Pts',(3.06703292504744,-8.38806678035338,108.681173529528));
#48324=CARTESIAN_POINT('Ctrl Pts',(2.675245980424,-8.40783455434159,108.541442708565));
#48325=CARTESIAN_POINT('Ctrl Pts',(2.57856569841362,-8.42760232832982,108.136875488718));
#48326=CARTESIAN_POINT('Ctrl Pts',(2.86484625061921,-8.44737010231804,107.835105447572));
#48327=CARTESIAN_POINT('Ctrl Pts',(3.27394213232089,-8.46713787630626,107.910353516512));
#48328=CARTESIAN_POINT('Ctrl Pts',(3.43410453346437,-8.48690565029448,108.294241153151));
#48329=CARTESIAN_POINT('Ctrl Pts',(3.19979255592849,-8.5066734242827,108.637926488142));
#48330=CARTESIAN_POINT('Ctrl Pts',(2.78392743096132,-8.52644119827092,108.629099816032));
#48331=CARTESIAN_POINT('Ctrl Pts',(2.56440923593972,-8.54620897225914,108.275782006746));
#48332=CARTESIAN_POINT('Ctrl Pts',(2.74071596962794,-8.56597674624737,107.899035874767));
#48333=CARTESIAN_POINT('Ctrl Pts',(3.15263624544216,-8.58574452023558,107.841213745114));
#48334=CARTESIAN_POINT('Ctrl Pts',(3.42585470304631,-8.60551229422381,108.154859065068));
#48335=CARTESIAN_POINT('Ctrl Pts',(3.31209547108053,-8.62528006821203,108.554959739207));
#48336=CARTESIAN_POINT('Ctrl Pts',(2.91473250417878,-8.64504784220024,108.677940976962));
#48337=CARTESIAN_POINT('Ctrl Pts',(2.59485281571043,-8.66481561618847,108.41204871079));
#48338=CARTESIAN_POINT('Ctrl Pts',(2.64313372331067,-8.68458339017669,107.998901441326));
#48339=CARTESIAN_POINT('Ctrl Pts',(3.01570196706283,-8.7043511641649,107.813929508179));
#48340=CARTESIAN_POINT('Ctrl Pts',(3.37400170352317,-8.72411893815313,108.025218436325));
#48341=CARTESIAN_POINT('Ctrl Pts',(3.39244299979417,-8.74388671214134,108.440768229847));
#48342=CARTESIAN_POINT('Ctrl Pts',(3.05426809748411,-8.76365448612957,108.68296535566));
#48343=CARTESIAN_POINT('Ctrl Pts',(2.66677932630862,-8.78342226011778,108.531723283083));
#48344=CARTESIAN_POINT('Ctrl Pts',(2.58209093634202,-8.80319003410601,108.124476933917));
#48345=CARTESIAN_POINT('Ctrl Pts',(2.87715996773966,-8.82295780809423,107.831294432709));
#48346=CARTESIAN_POINT('Ctrl Pts',(3.2838547520778,-8.84272558208245,107.918593142302));
#48347=CARTESIAN_POINT('Ctrl Pts',(3.43260837632838,-8.86249335607067,108.307044003515));
#48348=CARTESIAN_POINT('Ctrl Pts',(3.18824719225911,-8.8822611300589,108.643658507101));
#48349=CARTESIAN_POINT('Ctrl Pts',(2.77282422818049,-8.90202890404711,108.622552270567));
#48350=CARTESIAN_POINT('Ctrl Pts',(2.56383776621423,-8.92179667803534,108.262904705555));
#48351=CARTESIAN_POINT('Ctrl Pts',(2.75119553222219,-8.94156445202356,107.89153052791));
#48352=CARTESIAN_POINT('Ctrl Pts',(3.16464397518306,-8.96133222601178,107.845900523333));
#48353=CARTESIAN_POINT('Ctrl Pts',(3.42847907664,-8.9811,108.167479054246));
#48354=CARTESIAN_POINT('Ctrl Pts',(3.3029516985443,-9.00086777398822,108.564045050838));
#48355=CARTESIAN_POINT('Ctrl Pts',(2.90212960721617,-9.02063554797644,108.675235713249));
#48356=CARTESIAN_POINT('Ctrl Pts',(2.59024315098975,-9.04040332196466,108.400011167238));
#48357=CARTESIAN_POINT('Ctrl Pts',(2.6507061312773,-9.06017109595288,107.988470233284));
#48358=CARTESIAN_POINT('Ctrl Pts',(3.02857533798636,-9.0799388699411,107.81458356064));
#48359=CARTESIAN_POINT('Ctrl Pts',(3.3804778988175,-9.09970664392933,108.036363406408));
#48360=CARTESIAN_POINT('Ctrl Pts',(3.38663704723469,-9.11947441791755,108.452276591096));
#48361=CARTESIAN_POINT('Ctrl Pts',(3.04145591419998,-9.13924219190576,108.684379365051));
#48362=CARTESIAN_POINT('Ctrl Pts',(2.65860344910236,-9.15900996589399,108.521758018608));
#48363=CARTESIAN_POINT('Ctrl Pts',(2.58598085259615,-9.17877773988221,108.112187913759));
#48364=CARTESIAN_POINT('Ctrl Pts',(2.88958087802693,-9.19854551387043,107.82784879117));
#48365=CARTESIAN_POINT('Ctrl Pts',(3.29351967332174,-9.21831328785865,107.927121962161));
#48366=CARTESIAN_POINT('Ctrl Pts',(3.43073471295386,-9.23808106184687,108.319797076032));
#48367=CARTESIAN_POINT('Ctrl Pts',(3.17653756143592,-9.25784883583509,108.649047009009));
#48368=CARTESIAN_POINT('Ctrl Pts',(2.76191926004626,-9.27761660982331,108.615679627437));
#48369=CARTESIAN_POINT('Ctrl Pts',(2.56364691332878,-9.29738438381153,108.250016141092));
#48370=CARTESIAN_POINT('Ctrl Pts',(2.76189218531883,-9.31715215779975,107.884337995758));
#48371=CARTESIAN_POINT('Ctrl Pts',(3.17650808171374,-9.33691993178797,107.850939918326));
#48372=CARTESIAN_POINT('Ctrl Pts',(3.4307294408388,-9.35668770577619,108.180171077031));
#48373=CARTESIAN_POINT('Ctrl Pts',(3.2935437962731,-9.37645547976441,108.572856267372));
#48374=CARTESIAN_POINT('Ctrl Pts',(2.88961160504489,-9.39622325375264,108.672159490547));
#48375=CARTESIAN_POINT('Ctrl Pts',(2.58599215656126,-9.41599102774085,108.387842478632));
#48376=CARTESIAN_POINT('Ctrl Pts',(2.65858092553529,-9.43575880172908,107.978267781575));
#48377=CARTESIAN_POINT('Ctrl Pts',(3.04142899743941,-9.4555265757173,107.815616443488));
#48378=CARTESIAN_POINT('Ctrl Pts',(3.38661058630124,-9.47529434970552,108.047697417508));
#48379=CARTESIAN_POINT('Ctrl Pts',(3.38051827656907,-9.49506212369374,108.463603341592));
#48380=CARTESIAN_POINT('Ctrl Pts',(3.02855251802456,-9.51482989768196,108.685427531988));
#48381=CARTESIAN_POINT('Ctrl Pts',(2.65083971162567,-9.53459767167018,108.511534362189));
#48382=CARTESIAN_POINT('Ctrl Pts',(2.5899636169306,-9.5543654456584,108.100092074644));
#48383=CARTESIAN_POINT('Ctrl Pts',(2.90261527770578,-9.57413321964662,107.824706125944));
#48384=CARTESIAN_POINT('Ctrl Pts',(3.23500700524924,-9.59060636463681,107.917817535972));
#48385=CARTESIAN_POINT('Ctrl Pts',(3.36691627038736,-9.60378488062896,108.134169551681));
#48386=CARTESIAN_POINT('Ctrl Pts',(3.37453195781123,-9.61037413862503,108.259766361471));
#48387=CARTESIAN_POINT('Ctrl Pts',(3.36296026340509,-9.61366876762306,108.319874800994));
#48388=CARTESIAN_POINT('Ctrl Pts',(3.20090772186951,-7.72963123237693,107.968366390867));
#48389=CARTESIAN_POINT('Ctrl Pts',(3.24754797004252,-7.73292586137497,108.001637938381));
#48390=CARTESIAN_POINT('Ctrl Pts',(3.32345295254979,-7.73951511937104,108.091680985256));
#48391=CARTESIAN_POINT('Ctrl Pts',(3.3736919345866,-7.75269363536319,108.323462037814));
#48392=CARTESIAN_POINT('Ctrl Pts',(3.20850119787409,-7.76916678035338,108.601114506829));
#48393=CARTESIAN_POINT('Ctrl Pts',(2.81884242542315,-7.7889345543416,108.616264162071));
#48394=CARTESIAN_POINT('Ctrl Pts',(2.59453681216278,-7.80870232832982,108.298102620267));
#48395=CARTESIAN_POINT('Ctrl Pts',(2.73830465478089,-7.82847010231804,107.936444980801));
#48396=CARTESIAN_POINT('Ctrl Pts',(3.12003831607613,-7.84823787630626,107.859616651869));
#48397=CARTESIAN_POINT('Ctrl Pts',(3.39261509399311,-7.86800565029448,108.137578651642));
#48398=CARTESIAN_POINT('Ctrl Pts',(3.30845384589251,-7.8877734242827,108.517677687003));
#48399=CARTESIAN_POINT('Ctrl Pts',(2.94398191712845,-7.90754119827092,108.654545482088));
#48400=CARTESIAN_POINT('Ctrl Pts',(2.63042142278778,-7.92730897225914,108.423794989766));
#48401=CARTESIAN_POINT('Ctrl Pts',(2.65269664552128,-7.94707674624736,108.035117600806));
#48402=CARTESIAN_POINT('Ctrl Pts',(2.99057085101244,-7.96684452023558,107.841704682847));
#48403=CARTESIAN_POINT('Ctrl Pts',(3.33701268697619,-7.9866122942238,108.019313527799));
#48404=CARTESIAN_POINT('Ctrl Pts',(3.37720863610352,-8.00638006821202,108.406548878524));
#48405=CARTESIAN_POINT('Ctrl Pts',(3.07463182796275,-8.02614784220024,108.651527060338));
#48406=CARTESIAN_POINT('Ctrl Pts',(2.70423653002431,-8.04591561618847,108.531634240676));
#48407=CARTESIAN_POINT('Ctrl Pts',(2.60260391072527,-8.06568339017669,108.155818077281));
#48408=CARTESIAN_POINT('Ctrl Pts',(2.8620884180077,-8.0854511641649,107.865585796883));
#48409=CARTESIAN_POINT('Ctrl Pts',(3.24689431335474,-8.10521893815313,107.924673885216));
#48410=CARTESIAN_POINT('Ctrl Pts',(3.40734530795685,-8.12498671214135,108.279388501936));
#48411=CARTESIAN_POINT('Ctrl Pts',(3.1976382519198,-8.14475448612957,108.607397544827));
#48412=CARTESIAN_POINT('Ctrl Pts',(2.80833568296828,-8.16452226011779,108.610636483421));
#48413=CARTESIAN_POINT('Ctrl Pts',(2.59320006325944,-8.18429003410601,108.286162068016));
#48414=CARTESIAN_POINT('Ctrl Pts',(2.74772690957395,-8.20405780809423,107.928826882338));
#48415=CARTESIAN_POINT('Ctrl Pts',(3.13149639885665,-8.22382558208245,107.863344364136));
#48416=CARTESIAN_POINT('Ctrl Pts',(3.39577402333215,-8.24359335607067,108.149219019044));
#48417=CARTESIAN_POINT('Ctrl Pts',(3.30040852058379,-8.26336113005889,108.5266741846));
#48418=CARTESIAN_POINT('Ctrl Pts',(2.93205931144819,-8.28312890404711,108.652713231099));
#48419=CARTESIAN_POINT('Ctrl Pts',(2.62544836772165,-8.30289667803533,108.412803434919));
#48420=CARTESIAN_POINT('Ctrl Pts',(2.65919558899231,-8.32266445202356,108.02495281139));
#48421=CARTESIAN_POINT('Ctrl Pts',(3.00263459627197,-8.34243222601178,107.841604428812));
#48422=CARTESIAN_POINT('Ctrl Pts',(3.34367952413706,-8.3622,108.029368478334));
#48423=CARTESIAN_POINT('Ctrl Pts',(3.37242002692071,-8.38196777398822,108.417622215747));
#48424=CARTESIAN_POINT('Ctrl Pts',(3.06273937212083,-8.40173554797644,108.653556259832));
#48425=CARTESIAN_POINT('Ctrl Pts',(2.69604693115369,-8.42150332196466,108.522775394056));
#48426=CARTESIAN_POINT('Ctrl Pts',(2.60555915689196,-8.44127109595288,108.14412127243));
#48427=CARTESIAN_POINT('Ctrl Pts',(2.87350303794851,-8.46103886994111,107.861680025938));
#48428=CARTESIAN_POINT('Ctrl Pts',(3.25639575428181,-8.48080664392932,107.932108350456));
#48429=CARTESIAN_POINT('Ctrl Pts',(3.40629952885221,-8.50057441791754,108.291407445201));
#48430=CARTESIAN_POINT('Ctrl Pts',(3.18699556232252,-8.52034219190576,108.613079252141));
#48431=CARTESIAN_POINT('Ctrl Pts',(2.79776718225517,-8.54010996589398,108.604817940768));
#48432=CARTESIAN_POINT('Ctrl Pts',(2.5923094357074,-8.55987773988221,108.27413063303));
#48433=CARTESIAN_POINT('Ctrl Pts',(2.7573234756653,-8.57964551387043,107.921515619549));
#48434=CARTESIAN_POINT('Ctrl Pts',(3.14285967970434,-8.59941328785865,107.86739707845));
#48435=CARTESIAN_POINT('Ctrl Pts',(3.39857811165065,-8.61918106184687,108.160952975476));
#48436=CARTESIAN_POINT('Ctrl Pts',(3.2921053181476,-8.63894883583509,108.535426639916));
#48437=CARTESIAN_POINT('Ctrl Pts',(2.92019400695475,-8.65871660982331,108.650530756794));
#48438=CARTESIAN_POINT('Ctrl Pts',(2.62080306146777,-8.67848438381153,108.401669263437));
#48439=CARTESIAN_POINT('Ctrl Pts',(2.66599150917639,-8.69825215779975,108.014984656413));
#48440=CARTESIAN_POINT('Ctrl Pts',(3.01469623403554,-8.71801993178797,107.841860435183));
#48441=CARTESIAN_POINT('Ctrl Pts',(3.35004636952003,-8.73778770577619,108.039616010948));
#48442=CARTESIAN_POINT('Ctrl Pts',(3.36730647488344,-8.75755547976441,108.428549256992));
#48443=CARTESIAN_POINT('Ctrl Pts',(3.05079214967772,-8.77732325375264,108.655233316985));
#48444=CARTESIAN_POINT('Ctrl Pts',(2.68812257811692,-8.79709102774085,108.513678511417));
#48445=CARTESIAN_POINT('Ctrl Pts',(2.60885859838356,-8.81685880172908,108.132516862465));
#48446=CARTESIAN_POINT('Ctrl Pts',(2.88502804420571,-8.8366265757173,107.858113111926));
#48447=CARTESIAN_POINT('Ctrl Pts',(3.26567345683143,-8.85639434970552,107.93982021665));
#48448=CARTESIAN_POINT('Ctrl Pts',(3.40489920268056,-8.87616212369374,108.303390255031));
#48449=CARTESIAN_POINT('Ctrl Pts',(3.1761896953995,-8.89592989768196,108.618444127241));
#48450=CARTESIAN_POINT('Ctrl Pts',(2.78737515519524,-8.91569767167018,108.598689774779));
#48451=CARTESIAN_POINT('Ctrl Pts',(2.59177456941985,-8.9354654456584,108.262078141053));
#48452=CARTESIAN_POINT('Ctrl Pts',(2.76713180756785,-8.95523321964662,107.914491000691));
#48453=CARTESIAN_POINT('Ctrl Pts',(3.15409829750309,-8.97500099363484,107.871783661947));
#48454=CARTESIAN_POINT('Ctrl Pts',(3.40103439043249,-8.99476876762306,108.172764636635));
#48455=CARTESIAN_POINT('Ctrl Pts',(3.28354721707514,-9.01453654161128,108.543930024585));
#48456=CARTESIAN_POINT('Ctrl Pts',(2.90839834323012,-9.03430431559951,108.647998769019));
#48457=CARTESIAN_POINT('Ctrl Pts',(2.61648865224188,-9.05407208958772,108.390402741443));
#48458=CARTESIAN_POINT('Ctrl Pts',(2.67307889378527,-9.07383986357594,108.005221581886));
#48459=CARTESIAN_POINT('Ctrl Pts',(3.0267450474843,-9.09360763756417,107.842472594666));
#48460=CARTESIAN_POINT('Ctrl Pts',(3.35610775541675,-9.11337541155239,108.050047130056));
#48461=CARTESIAN_POINT('Ctrl Pts',(3.36187240173376,-9.13314318554061,108.439320491552));
#48462=CARTESIAN_POINT('Ctrl Pts',(3.03880060471419,-9.15291095952883,108.65655675709));
#48463=CARTESIAN_POINT('Ctrl Pts',(2.68047037732015,-9.17267873351705,108.504351536118));
#48464=CARTESIAN_POINT('Ctrl Pts',(2.61249936004231,-9.19244650750527,108.121014971295));
#48465=CARTESIAN_POINT('Ctrl Pts',(2.89665337775696,-9.21221428149349,107.854888168563));
#48466=CARTESIAN_POINT('Ctrl Pts',(3.27471932630547,-9.23198205548171,107.947802753628));
#48467=CARTESIAN_POINT('Ctrl Pts',(3.40314555007477,-9.25174982946993,108.315326475355));
#48468=CARTESIAN_POINT('Ctrl Pts',(3.16523008286441,-9.27151760345816,108.62348748804));
#48469=CARTESIAN_POINT('Ctrl Pts',(2.77716866557457,-9.29128537744637,108.592257334087));
#48470=CARTESIAN_POINT('Ctrl Pts',(2.59159594092957,-9.3110531514346,108.250015107232));
#48471=CARTESIAN_POINT('Ctrl Pts',(2.77714332502144,-9.33082092542281,107.907759160318));
#48472=CARTESIAN_POINT('Ctrl Pts',(3.16520249135981,-9.35058869941103,107.876500276617));
#48473=CARTESIAN_POINT('Ctrl Pts',(3.40314061564608,-9.37035647339926,108.184643717548));
#48474=CARTESIAN_POINT('Ctrl Pts',(3.27474190414793,-9.39012424738748,108.552176870334));
#48475=CARTESIAN_POINT('Ctrl Pts',(2.89668213666629,-9.4098920213757,108.645119582698));
#48476=CARTESIAN_POINT('Ctrl Pts',(2.61250993997259,-9.42965979536392,108.37901347442));
#48477=CARTESIAN_POINT('Ctrl Pts',(2.68044929641917,-9.44942756935214,107.995672611527));
#48478=CARTESIAN_POINT('Ctrl Pts',(3.03877541200992,-9.46919534334036,107.843439319918));
#48479=CARTESIAN_POINT('Ctrl Pts',(3.36184763566024,-9.48896311732858,108.060655181838));
#48480=CARTESIAN_POINT('Ctrl Pts',(3.35614554691665,-9.5087308913168,108.449921747782));
#48481=CARTESIAN_POINT('Ctrl Pts',(3.02672368917307,-9.52849866530503,108.657537787464));
#48482=CARTESIAN_POINT('Ctrl Pts',(2.67320391812486,-9.54826643929324,108.49478271924));
#48483=CARTESIAN_POINT('Ctrl Pts',(2.61622702273152,-9.56803421328147,108.109693887651));
#48484=CARTESIAN_POINT('Ctrl Pts',(2.90885290584327,-9.58780198726969,107.851946795456));
#48485=CARTESIAN_POINT('Ctrl Pts',(3.21995447674257,-9.60427513225987,107.939094288995));
#48486=CARTESIAN_POINT('Ctrl Pts',(3.34341476832062,-9.61745364825202,108.141588654458));
#48487=CARTESIAN_POINT('Ctrl Pts',(3.35054266027676,-9.62404290624809,108.259140812312));
#48488=CARTESIAN_POINT('Ctrl Pts',(3.33971214913761,-9.62733753524613,108.315399221924));
#48489=CARTESIAN_POINT('Ctrl Pts',(3.18715865317386,-7.7433,107.987639915065));
#48490=CARTESIAN_POINT('Ctrl Pts',(3.23060708786083,-7.74659462899803,108.018634532712));
#48491=CARTESIAN_POINT('Ctrl Pts',(3.30131753225317,-7.75318388699411,108.102515506643));
#48492=CARTESIAN_POINT('Ctrl Pts',(3.34811842236999,-7.76636240298626,108.318434681996));
#48493=CARTESIAN_POINT('Ctrl Pts',(3.19423247158511,-7.78283554797644,108.577086075122));
#48494=CARTESIAN_POINT('Ctrl Pts',(2.83123989782698,-7.80260332196466,108.591198967572));
#48495=CARTESIAN_POINT('Ctrl Pts',(2.62228458199092,-7.82237109595288,108.294810729719));
#48496=CARTESIAN_POINT('Ctrl Pts',(2.75621370897387,-7.8421388699411,107.957903038554));
#48497=CARTESIAN_POINT('Ctrl Pts',(3.1118235245366,-7.86190664392932,107.886332436713));
#48498=CARTESIAN_POINT('Ctrl Pts',(3.3657465801897,-7.88167441791754,108.145272177939));
#48499=CARTESIAN_POINT('Ctrl Pts',(3.28734488563378,-7.90144219190576,108.499359232776));
#48500=CARTESIAN_POINT('Ctrl Pts',(2.94781550033985,-7.92120996589399,108.626860515219));
#48501=CARTESIAN_POINT('Ctrl Pts',(2.65571343844177,-7.9409777398822,108.411901373976));
#48502=CARTESIAN_POINT('Ctrl Pts',(2.6764642619898,-7.96074551387043,108.04982302298));
#48503=CARTESIAN_POINT('Ctrl Pts',(2.99121613241808,-7.98051328785865,107.869646268722));
#48504=CARTESIAN_POINT('Ctrl Pts',(3.31394930971311,-8.00028106184687,108.035100497677));
#48505=CARTESIAN_POINT('Ctrl Pts',(3.35139445931568,-8.02004883583509,108.395835495957));
#48506=CARTESIAN_POINT('Ctrl Pts',(3.0695244178543,-8.03981660982331,108.624048658391));
#48507=CARTESIAN_POINT('Ctrl Pts',(2.72447702764442,-8.05958438381153,108.512360673259));
#48508=CARTESIAN_POINT('Ctrl Pts',(2.62979961072117,-8.07935215779975,108.162263393137));
#48509=CARTESIAN_POINT('Ctrl Pts',(2.87152636194084,-8.09911993178797,107.891893084811));
#48510=CARTESIAN_POINT('Ctrl Pts',(3.22999816400173,-8.11888770577619,107.946937494892));
#48511=CARTESIAN_POINT('Ctrl Pts',(3.37946873571844,-8.13865547976441,108.277377307303));
#48512=CARTESIAN_POINT('Ctrl Pts',(3.18411292856613,-8.15842325375263,108.582939135017));
#48513=CARTESIAN_POINT('Ctrl Pts',(2.8214521816118,-8.17819102774085,108.585956417675));
#48514=CARTESIAN_POINT('Ctrl Pts',(2.62103931315779,-8.19795880172907,108.283687326116));
#48515=CARTESIAN_POINT('Ctrl Pts',(2.76499115416374,-8.2177265757173,107.950806282716));
#48516=CARTESIAN_POINT('Ctrl Pts',(3.12249747634493,-8.23749434970551,107.889805043942));
#48517=CARTESIAN_POINT('Ctrl Pts',(3.36868932900526,-8.25726212369374,108.156115939767));
#48518=CARTESIAN_POINT('Ctrl Pts',(3.27985014011025,-8.27702989768196,108.507740057355));
#48519=CARTESIAN_POINT('Ctrl Pts',(2.93670881513792,-8.29679767167018,108.625153653859));
#48520=CARTESIAN_POINT('Ctrl Pts',(2.65108071313049,-8.3165654456584,108.401662023381));
#48521=CARTESIAN_POINT('Ctrl Pts',(2.68251845192224,-8.33633321964662,108.040353858334));
#48522=CARTESIAN_POINT('Ctrl Pts',(3.00245429834817,-8.35610099363484,107.869552875547));
#48523=CARTESIAN_POINT('Ctrl Pts',(3.32015990357356,-8.37586876762306,108.044467340237));
#48524=CARTESIAN_POINT('Ctrl Pts',(3.34693355738075,-8.39563654161128,108.406151032172));
#48525=CARTESIAN_POINT('Ctrl Pts',(3.05844581919422,-8.4154043155995,108.625938990135));
#48526=CARTESIAN_POINT('Ctrl Pts',(2.71684788188338,-8.43517208958773,108.504108079548));
#48527=CARTESIAN_POINT('Ctrl Pts',(2.63255261537031,-8.45493986357594,108.151367056142));
#48528=CARTESIAN_POINT('Ctrl Pts',(2.8821598252778,-8.47470763756417,107.888254604305));
#48529=CARTESIAN_POINT('Ctrl Pts',(3.23884937624272,-8.49447541155238,107.9538631844));
#48530=CARTESIAN_POINT('Ctrl Pts',(3.37849452424005,-8.51424318554061,108.288573737252));
#48531=CARTESIAN_POINT('Ctrl Pts',(3.17419856871655,-8.53401095952883,108.58823201614));
#48532=CARTESIAN_POINT('Ctrl Pts',(2.81160693354902,-8.55377873351705,108.580536065503));
#48533=CARTESIAN_POINT('Ctrl Pts',(2.62020963547507,-8.57354650750527,108.272479259314));
#48534=CARTESIAN_POINT('Ctrl Pts',(2.77393098170266,-8.59331428149349,107.94399536433));
#48535=CARTESIAN_POINT('Ctrl Pts',(3.13308311396652,-8.61308205548171,107.893580411787));
#48536=CARTESIAN_POINT('Ctrl Pts',(3.37130152025498,-8.63284982946993,108.167046885883));
#48537=CARTESIAN_POINT('Ctrl Pts',(3.27211516521468,-8.65261760345815,108.515893540624));
#48538=CARTESIAN_POINT('Ctrl Pts',(2.92565550973071,-8.67238537744637,108.623120536626));
#48539=CARTESIAN_POINT('Ctrl Pts',(2.6467533072251,-8.6921531514346,108.391289816083));
#48540=CARTESIAN_POINT('Ctrl Pts',(2.68884929504212,-8.71192092542282,108.0310678715));
#48541=CARTESIAN_POINT('Ctrl Pts',(3.01369050100825,-8.73168869941104,107.869791362187));
#48542=CARTESIAN_POINT('Ctrl Pts',(3.32609103551689,-8.75145647339926,108.054013585571));
#48543=CARTESIAN_POINT('Ctrl Pts',(3.34216994997271,-8.77122424738748,108.416330284137));
#48544=CARTESIAN_POINT('Ctrl Pts',(3.04731620187133,-8.7909920213757,108.62750127831));
#48545=CARTESIAN_POINT('Ctrl Pts',(2.70946582992522,-8.81075979536392,108.495633739751));
#48546=CARTESIAN_POINT('Ctrl Pts',(2.6356262604251,-8.83052756935215,108.140556791013));
#48547=CARTESIAN_POINT('Ctrl Pts',(2.89289612067176,-8.85029534334036,107.884931791143));
#48548=CARTESIAN_POINT('Ctrl Pts',(3.24749216158505,-8.87006311732858,107.961047290999));
#48549=CARTESIAN_POINT('Ctrl Pts',(3.37719002903275,-8.88983089131681,108.299736506548));
#48550=CARTESIAN_POINT('Ctrl Pts',(3.16413219853988,-8.90959866530502,108.593229747382));
#48551=CARTESIAN_POINT('Ctrl Pts',(2.80192608220999,-8.92936643929325,108.574827278991));
#48552=CARTESIAN_POINT('Ctrl Pts',(2.61971137262547,-8.94913421328146,108.261251576551));
#48553=CARTESIAN_POINT('Ctrl Pts',(2.78306808291351,-8.96890198726969,107.937451473473));
#48554=CARTESIAN_POINT('Ctrl Pts',(3.14355261982312,-8.9886697612579,107.897666800561));
#48555=CARTESIAN_POINT('Ctrl Pts',(3.37358970422498,-9.00843753524613,108.178050219025));
#48556=CARTESIAN_POINT('Ctrl Pts',(3.26414273560599,-9.02820530923435,108.523814998333));
#48557=CARTESIAN_POINT('Ctrl Pts',(2.91466707924407,-9.04797308322257,108.620761824788));
#48558=CARTESIAN_POINT('Ctrl Pts',(2.64273415349401,-9.06774085721079,108.380794315648));
#48559=CARTESIAN_POINT('Ctrl Pts',(2.69545165629325,-9.08750863119901,108.021972930488));
#48560=CARTESIAN_POINT('Ctrl Pts',(3.02491475698223,-9.10727640518723,107.870361628692));
#48561=CARTESIAN_POINT('Ctrl Pts',(3.331737612016,-9.12704417917545,108.063730853703));
#48562=CARTESIAN_POINT('Ctrl Pts',(3.33710775623283,-9.14681195316367,108.426364392007));
#48563=CARTESIAN_POINT('Ctrl Pts',(3.0361452952284,-9.1665797271519,108.628734149129));
#48564=CARTESIAN_POINT('Ctrl Pts',(2.70233730553794,-9.18634750114011,108.486945053627));
#48565=CARTESIAN_POINT('Ctrl Pts',(2.63901786748847,-9.20611527512833,108.129842028831));
#48566=CARTESIAN_POINT('Ctrl Pts',(2.90372587748699,-9.22588304911656,107.881927545957));
#48567=CARTESIAN_POINT('Ctrl Pts',(3.25591897928919,-9.24565082310478,107.968483545095));
#48568=CARTESIAN_POINT('Ctrl Pts',(3.37555638719568,-9.265418597093,108.310855874679));
#48569=CARTESIAN_POINT('Ctrl Pts',(3.15392260429289,-9.28518637108122,108.597927967071));
#48570=CARTESIAN_POINT('Ctrl Pts',(2.79241807110289,-9.30495414506944,108.568835040736));
#48571=CARTESIAN_POINT('Ctrl Pts',(2.61954496853035,-9.32472191905766,108.250014073372));
#48572=CARTESIAN_POINT('Ctrl Pts',(2.79239446472405,-9.34448969304588,107.931180324878));
#48573=CARTESIAN_POINT('Ctrl Pts',(3.15389690100588,-9.3642574670341,107.902060634909));
#48574=CARTESIAN_POINT('Ctrl Pts',(3.37555179045336,-9.38402524102232,108.189116358066));
#48575=CARTESIAN_POINT('Ctrl Pts',(3.25594001202276,-9.40379301501054,108.531497473297));
#48576=CARTESIAN_POINT('Ctrl Pts',(2.9037526682877,-9.42356078899877,108.618079674849));
#48577=CARTESIAN_POINT('Ctrl Pts',(2.63902772338391,-9.44332856298698,108.370184470209));
#48578=CARTESIAN_POINT('Ctrl Pts',(2.70231766730304,-9.46309633697521,108.01307744148));
#48579=CARTESIAN_POINT('Ctrl Pts',(3.03612182658042,-9.48286411096343,107.871262196348));
#48580=CARTESIAN_POINT('Ctrl Pts',(3.33708468501923,-9.50263188495165,108.073612946168));
#48581=CARTESIAN_POINT('Ctrl Pts',(3.33177281726424,-9.52239965893987,108.436240153971));
#48582=CARTESIAN_POINT('Ctrl Pts',(3.02489486032158,-9.54216743292809,108.629648042939));
#48583=CARTESIAN_POINT('Ctrl Pts',(2.69556812462404,-9.56193520691631,108.478031076292));
#48584=CARTESIAN_POINT('Ctrl Pts',(2.64249042853245,-9.58170298090453,108.119295700658));
#48585=CARTESIAN_POINT('Ctrl Pts',(2.91509053398075,-9.60147075489276,107.879187464968));
#48586=CARTESIAN_POINT('Ctrl Pts',(3.20490194823591,-9.61794389988293,107.960371042017));
#48587=CARTESIAN_POINT('Ctrl Pts',(3.31991326625387,-9.63112241587508,108.149007757235));
#48588=CARTESIAN_POINT('Ctrl Pts',(3.32655336274228,-9.63771167387116,108.258515263153));
#48589=CARTESIAN_POINT('Ctrl Pts',(3.31646403487013,-9.64100630286919,108.310923642855));
#48590=CARTESIAN_POINT('',(3.38620837767256,-9.6,108.324350380063));
#48591=CARTESIAN_POINT('Ctrl Pts',(2.9047663113757,-9.6,107.941669514675));
#48592=CARTESIAN_POINT('Ctrl Pts',(2.91208752841734,-9.6,107.938464535723));
#48593=CARTESIAN_POINT('Ctrl Pts',(2.91951909466324,-9.6,107.93555598867));
#48594=CARTESIAN_POINT('Ctrl Pts',(2.9270473341129,-9.6,107.93295579821));
#48595=CARTESIAN_POINT('Ctrl Pts',(2.94169878127661,-9.6,107.927895311836));
#48596=CARTESIAN_POINT('Ctrl Pts',(2.95671562307874,-9.6,107.924001174705));
#48597=CARTESIAN_POINT('Ctrl Pts',(2.97197926144626,-9.6,107.921221613959));
#48598=CARTESIAN_POINT('Ctrl Pts',(2.98074175619374,-9.6,107.9196259337));
#48599=CARTESIAN_POINT('Ctrl Pts',(2.98959245259031,-9.6,107.918397815162));
#48600=CARTESIAN_POINT('Ctrl Pts',(2.998474281856,-9.6,107.917533107911));
#48601=CARTESIAN_POINT('Ctrl Pts',(3.01468072942063,-9.6,107.915955298622));
#48602=CARTESIAN_POINT('Ctrl Pts',(3.03100700663023,-9.6,107.915581069742));
#48603=CARTESIAN_POINT('Ctrl Pts',(3.04732282720845,-9.6,107.916357855643));
#48604=CARTESIAN_POINT('Ctrl Pts',(3.0550860205024,-9.6,107.916727456368));
#48605=CARTESIAN_POINT('Ctrl Pts',(3.06284700521599,-9.6,107.917358017175));
#48606=CARTESIAN_POINT('Ctrl Pts',(3.07059229349538,-9.6,107.918245921928));
#48607=CARTESIAN_POINT('Ctrl Pts',(3.07645289849991,-9.6,107.918917770264));
#48608=CARTESIAN_POINT('Ctrl Pts',(3.08229730575072,-9.6,107.919736283014));
#48609=CARTESIAN_POINT('Ctrl Pts',(3.08811244646604,-9.6,107.92069772171));
#48610=CARTESIAN_POINT('Ctrl Pts',(3.10788527884949,-9.6,107.92396683713));
#48611=CARTESIAN_POINT('Ctrl Pts',(3.1273446475303,-9.6,107.928887258058));
#48612=CARTESIAN_POINT('Ctrl Pts',(3.14626667162367,-9.6,107.935377526743));
#48613=CARTESIAN_POINT('Ctrl Pts',(3.15848777788601,-9.6,107.939569375505));
#48614=CARTESIAN_POINT('Ctrl Pts',(3.17048510749447,-9.6,107.944417154964));
#48615=CARTESIAN_POINT('Ctrl Pts',(3.18219822161691,-9.6,107.949910387659));
#48616=CARTESIAN_POINT('Ctrl Pts',(3.18735667522611,-9.6,107.95232960647));
#48617=CARTESIAN_POINT('Ctrl Pts',(3.19245998065074,-9.6,107.954874127728));
#48618=CARTESIAN_POINT('Ctrl Pts',(3.19750279605545,-9.6,107.957543597182));
#48619=CARTESIAN_POINT('Ctrl Pts',(3.20191914257529,-9.6,107.959881438485));
#48620=CARTESIAN_POINT('Ctrl Pts',(3.20628611153622,-9.6,107.962313705682));
#48621=CARTESIAN_POINT('Ctrl Pts',(3.21059155521031,-9.6,107.964834412739));
#48622=CARTESIAN_POINT('Ctrl Pts',(3.22417397784133,-9.6,107.9727865104));
#48623=CARTESIAN_POINT('Ctrl Pts',(3.2371700909409,-9.6,107.981630931996));
#48624=CARTESIAN_POINT('Ctrl Pts',(3.24947753805501,-9.6,107.991337449338));
#48625=CARTESIAN_POINT('Ctrl Pts',(3.26144617364877,-9.6,108.000776756114));
#48626=CARTESIAN_POINT('Ctrl Pts',(3.27276398520879,-9.6,108.011031382882));
#48627=CARTESIAN_POINT('Ctrl Pts',(3.28339510187528,-9.6,108.02200369201));
#48628=CARTESIAN_POINT('Ctrl Pts',(3.2894425301682,-9.6,108.02824520499));
#48629=CARTESIAN_POINT('Ctrl Pts',(3.29526760808024,-9.6,108.034719247612));
#48630=CARTESIAN_POINT('Ctrl Pts',(3.3008622810014,-9.6,108.041409871992));
#48631=CARTESIAN_POINT('Ctrl Pts',(3.30502766752572,-9.6,108.046391224258));
#48632=CARTESIAN_POINT('Ctrl Pts',(3.30906699199165,-9.6,108.051495376588));
#48633=CARTESIAN_POINT('Ctrl Pts',(3.31296183144936,-9.6,108.056695204982));
#48634=CARTESIAN_POINT('Ctrl Pts',(3.32548548455846,-9.6,108.07341498194));
#48635=CARTESIAN_POINT('Ctrl Pts',(3.33655220478908,-9.6,108.091159138622));
#48636=CARTESIAN_POINT('Ctrl Pts',(3.34607870297481,-9.6,108.109684473486));
#48637=CARTESIAN_POINT('Ctrl Pts',(3.35059666448507,-9.6,108.118470151944));
#48638=CARTESIAN_POINT('Ctrl Pts',(3.35476778148254,-9.6,108.127432195746));
#48639=CARTESIAN_POINT('Ctrl Pts',(3.35858042570842,-9.6,108.136547646305));
#48640=CARTESIAN_POINT('Ctrl Pts',(3.36323661049533,-9.6,108.147679873628));
#48641=CARTESIAN_POINT('Ctrl Pts',(3.36735832511144,-9.6,108.159040884373));
#48642=CARTESIAN_POINT('Ctrl Pts',(3.37093902375822,-9.6,108.170594501883));
#48643=CARTESIAN_POINT('Ctrl Pts',(3.3725349679066,-9.6,108.175744035556));
#48644=CARTESIAN_POINT('Ctrl Pts',(3.37402327625765,-9.6,108.180932309664));
#48645=CARTESIAN_POINT('Ctrl Pts',(3.37539961282126,-9.6,108.18614094522));
#48646=CARTESIAN_POINT('Ctrl Pts',(3.38089186464593,-9.6,108.206925932622));
#48647=CARTESIAN_POINT('Ctrl Pts',(3.38462307558806,-9.6,108.228089606938));
#48648=CARTESIAN_POINT('Ctrl Pts',(3.38659117017677,-9.6,108.249415616141));
#48649=CARTESIAN_POINT('Ctrl Pts',(3.38856090362137,-9.6,108.270759383766));
#48650=CARTESIAN_POINT('Ctrl Pts',(3.38876502618137,-9.6,108.292267093563));
#48651=CARTESIAN_POINT('Ctrl Pts',(3.38715357967984,-9.6,108.313739432014));
#48652=CARTESIAN_POINT('Ctrl Pts',(3.38688804448339,-9.6,108.317277657828));
#48653=CARTESIAN_POINT('Ctrl Pts',(3.38657309767225,-9.6,108.320814935752));
#48654=CARTESIAN_POINT('Ctrl Pts',(3.38620837767256,-9.6,108.324350380063));
#48655=CARTESIAN_POINT('Ctrl Pts',(3.38620837767256,-9.6,108.324350380063));
#48656=CARTESIAN_POINT('Ctrl Pts',(3.39852125534571,-9.59670537100196,108.26039191063));
#48657=CARTESIAN_POINT('Ctrl Pts',(3.39446951389991,-9.59341074200393,108.193571179767));
#48658=CARTESIAN_POINT('Ctrl Pts',(3.37489886333973,-9.59011611300589,108.131384606091));
#48659=CARTESIAN_POINT('Ctrl Pts',(3.35532821277956,-9.58682148400785,108.069198032416));
#48660=CARTESIAN_POINT('Ctrl Pts',(3.320238653105,-9.58352685500982,108.011645615927));
#48661=CARTESIAN_POINT('Ctrl Pts',(3.2732668210428,-9.58023222601178,107.9666723165));
#48662=CARTESIAN_POINT('Ctrl Pts',(3.17932315691838,-9.5736429680157,107.876725717647));
#48663=CARTESIAN_POINT('Ctrl Pts',(3.03785040324334,-9.56705371001963,107.83709558704));
#48664=CARTESIAN_POINT('Ctrl Pts',(2.91166778666605,-9.56046445202356,107.86611798927));
#48665=CARTESIAN_POINT('Ctrl Pts',(2.78548517008876,-9.55387519402749,107.895140391501));
#48666=CARTESIAN_POINT('Ctrl Pts',(2.67459269060921,-9.54728593603141,107.992815326569));
#48667=CARTESIAN_POINT('Ctrl Pts',(2.62994233320224,-9.54069667803534,108.114618751353));
#48668=CARTESIAN_POINT('Ctrl Pts',(2.61417555827885,-9.53836990275806,108.157629542195));
#48669=CARTESIAN_POINT('Ctrl Pts',(2.60666859404062,-9.53604312748078,108.203648943736));
#48670=CARTESIAN_POINT('Ctrl Pts',(2.60697877099099,-9.5337163522035,108.249759674367));
#48671=CARTESIAN_POINT('Origin',(3.35,-7.7,108.25));
#48672=CARTESIAN_POINT('',(2.65,-7.7,108.25));
#48673=CARTESIAN_POINT('Origin',(3.,-7.7,108.25));
#48674=CARTESIAN_POINT('Origin',(3.,-7.725,108.25));
#48675=CARTESIAN_POINT('',(2.625,-7.725,108.25));
#48676=CARTESIAN_POINT('Origin',(3.,-8.675,108.25));
#48677=CARTESIAN_POINT('Origin',(3.,-9.6,108.25));
#48678=CARTESIAN_POINT('Origin',(3.9,-9.6,108.25));
#48679=CARTESIAN_POINT('',(2.1,-9.6,108.25));
#48680=CARTESIAN_POINT('Origin',(3.,-9.6,108.25));
#48681=CARTESIAN_POINT('Origin',(3.,-9.7,108.25));
#48682=CARTESIAN_POINT('',(2.,-9.7,108.25));
#48683=CARTESIAN_POINT('Origin',(3.,-11.1,108.25));
#48684=CARTESIAN_POINT('',(2.,-11.2,108.25));
#48685=CARTESIAN_POINT('Origin',(3.,-11.2,108.25));
#48686=CARTESIAN_POINT('',(1.95,-11.1,108.25));
#48687=CARTESIAN_POINT('Origin',(3.,-11.2,108.25));
#71458=UNCERTAINTY_MEASURE_WITH_UNIT(LENGTH_MEASURE(0.001),#71493,
'DISTANCE_ACCURACY_VALUE',
'Maximum model space distance between geometric entities at asserted c
onnectivities');
#71471=UNCERTAINTY_MEASURE_WITH_UNIT(LENGTH_MEASURE(0.001),#71493,
'DISTANCE_ACCURACY_VALUE',
'Maximum model space distance between geometric entities at asserted c
onnectivities');
#71479=(
GEOMETRIC_REPRESENTATION_CONTEXT(3)
GLOBAL_UNCERTAINTY_ASSIGNED_CONTEXT((#71458))
GLOBAL_UNIT_ASSIGNED_CONTEXT((#71493,#71495,#71496))
REPRESENTATION_CONTEXT('','3D')
);
#71492=(
GEOMETRIC_REPRESENTATION_CONTEXT(3)
GLOBAL_UNCERTAINTY_ASSIGNED_CONTEXT((#71471))
GLOBAL_UNIT_ASSIGNED_CONTEXT((#71493,#71495,#71496))
REPRESENTATION_CONTEXT('','3D')
);
#71493=(
LENGTH_UNIT()
NAMED_UNIT(*)
SI_UNIT(.CENTI.,.METRE.)
);
#71495=(
NAMED_UNIT(*)
PLANE_ANGLE_UNIT()
SI_UNIT($,.RADIAN.)
);
#71496=(
NAMED_UNIT(*)
SI_UNIT($,.STERADIAN.)
SOLID_ANGLE_UNIT()
);
#71504=SHAPE_DEFINITION_REPRESENTATION(#71524,#71609);
#71524=PRODUCT_DEFINITION_SHAPE('',$,#71630);
#71609=SHAPE_REPRESENTATION('',(#29736),#71479);
#71622=PRODUCT_DEFINITION_CONTEXT('part definition',#71684,'design');
#71630=PRODUCT_DEFINITION('2026-10-19-03-22-35-930',
'12_Hydraulic_Release_Valve_Knob_M8',#71650,#71622);
#71650=PRODUCT_DEFINITION_FORMATION('',$,#71693);
#71684=APPLICATION_CONTEXT(
'Core Data for Automotive Mechanical Design Process');
#71685=PRODUCT_CONTEXT('part definition',#71684,'mechanical');
#71693=PRODUCT('2026-10-19-03-22-35-930',
'12_Hydraulic_Release_Valve_Knob_M8',$,(#71685));
#71867=COLOUR_RGB('Light Blue',0.38,0.62,0.78);
#71868=FILL_AREA_STYLE_COLOUR('',#71867);
#71869=FILL_AREA_STYLE('',(#71868));
#71870=SURFACE_STYLE_FILL_AREA(#71869);
#71871=SURFACE_SIDE_STYLE('',(#71870));
#71872=SURFACE_STYLE_USAGE(.BOTH.,#71871);
#71873=PRESENTATION_STYLE_ASSIGNMENT((#71872));
ENDSEC;
END-ISO-10303-21;
